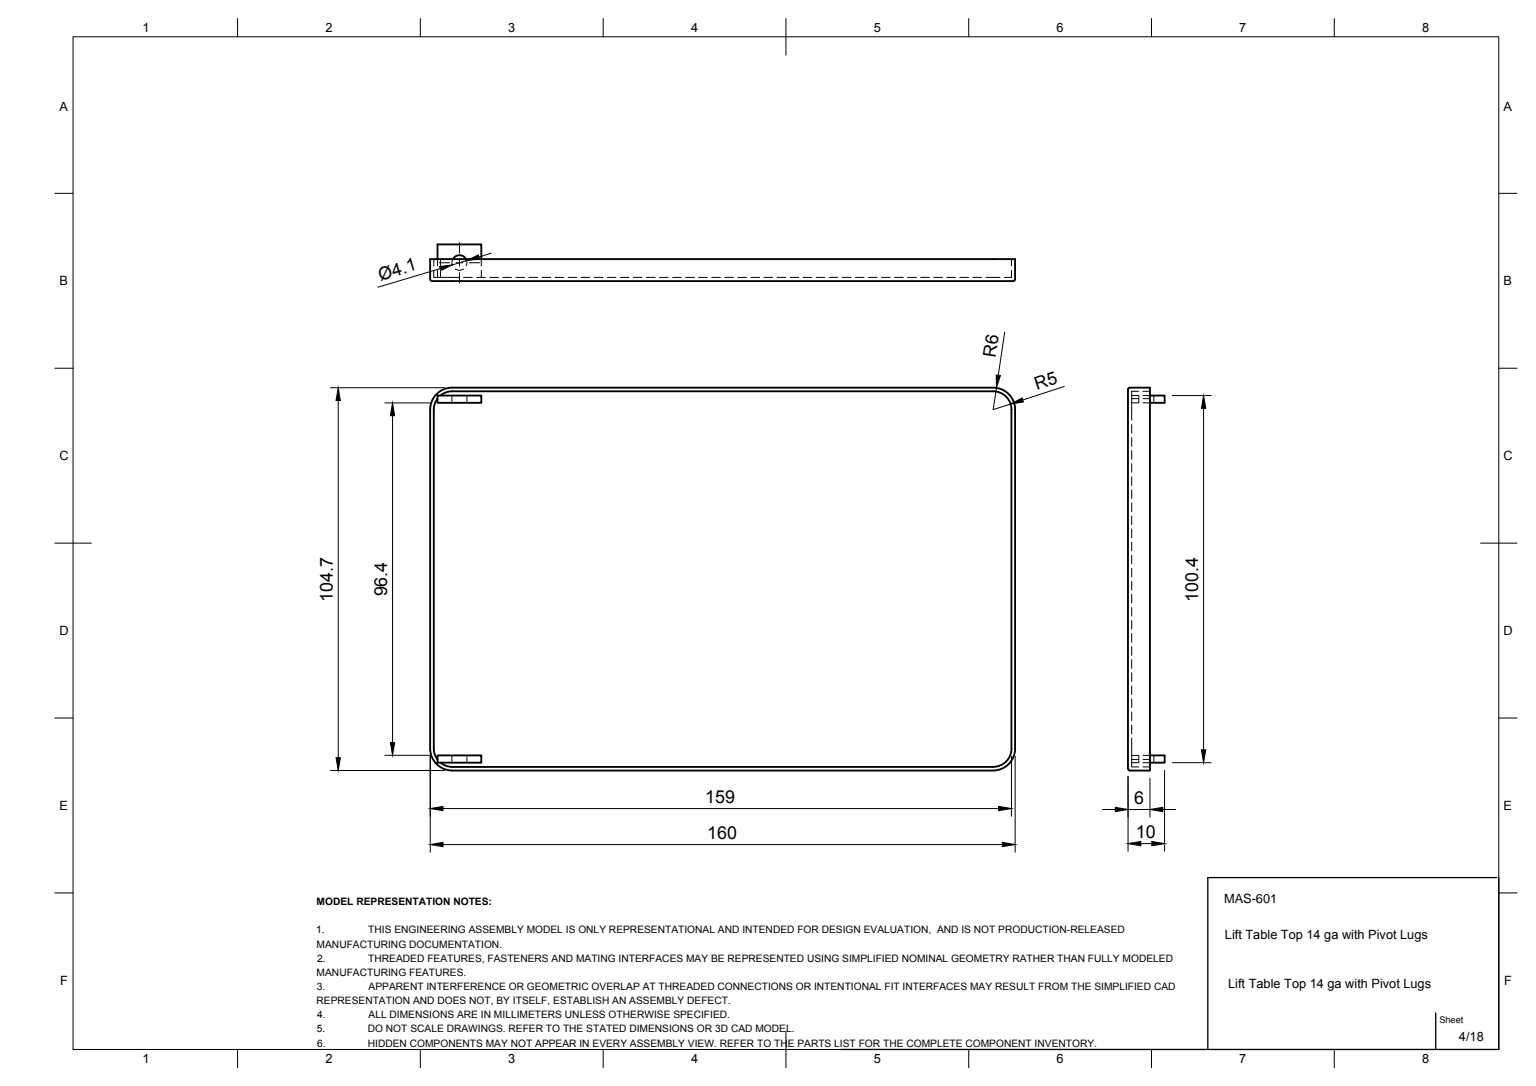
ISO-10303-21;
HEADER;
FILE_DESCRIPTION((''),'2;1');
FILE_NAME('Lift Table Top 14 ga with Pivot Lugs.step','2026-10-06T07:37:42+05:00',(''),(''),'','','');
FILE_SCHEMA (('AUTOMOTIVE_DESIGN { 1 0 10303 214 3 1 1 }'));
ENDSEC;
DATA;
#10=MECHANICAL_DESIGN_GEOMETRIC_PRESENTATION_REPRESENTATION('',(#374),#18757);
#331=TOROIDAL_SURFACE('',#9944,5.50000000000001,0.5) ;
#332=TOROIDAL_SURFACE('',#9950,5.50000000000001,0.5) ;
#333=TOROIDAL_SURFACE('',#9956,5.50000000000001,0.5) ;
#334=TOROIDAL_SURFACE('',#9962,5.50000000000001,0.5) ;
#340=SHAPE_REPRESENTATION_RELATIONSHIP('SRR','None',#18858,#357) ;
#357=ADVANCED_BREP_SHAPE_REPRESENTATION('',(#391),#18741) ;
#374=STYLED_ITEM('',(#18952),#391) ;
#391=MANIFOLD_SOLID_BREP('Lift Table Top 14 ga with Pivot Lugs',#9543) ;
#522=CYLINDRICAL_SURFACE('',#9906,2.05) ;
#523=CYLINDRICAL_SURFACE('',#9909,2.05) ;
#524=CYLINDRICAL_SURFACE('',#9917,5.00000000000001) ;
#525=CYLINDRICAL_SURFACE('',#9920,5.00000000000001) ;
#526=CYLINDRICAL_SURFACE('',#9937,5.00000000000001) ;
#527=CYLINDRICAL_SURFACE('',#9939,5.00000000000001) ;
#528=CYLINDRICAL_SURFACE('',#9941,0.5) ;
#529=CYLINDRICAL_SURFACE('',#9948,0.5) ;
#530=CYLINDRICAL_SURFACE('',#9954,0.5) ;
#531=CYLINDRICAL_SURFACE('',#9960,0.5) ;
#532=CYLINDRICAL_SURFACE('',#9965,6.00000000000001) ;
#533=CYLINDRICAL_SURFACE('',#9967,6.00000000000001) ;
#534=CYLINDRICAL_SURFACE('',#9971,5.00000000000001) ;
#535=CYLINDRICAL_SURFACE('',#9976,5.00000000000001) ;
#536=CYLINDRICAL_SURFACE('',#9979,6.00000000000001) ;
#537=CYLINDRICAL_SURFACE('',#9981,6.00000000000001) ;
#677=FACE_BOUND('',#1733,.T.) ;
#678=FACE_BOUND('',#1738,.T.) ;
#679=FACE_BOUND('',#1742,.T.) ;
#680=FACE_BOUND('',#1744,.T.) ;
#681=FACE_BOUND('',#1747,.T.) ;
#819=PLANE('',#9912) ;
#820=PLANE('',#9913) ;
#821=PLANE('',#9914) ;
#822=PLANE('',#9915) ;
#823=PLANE('',#9916) ;
#824=PLANE('',#9923) ;
#825=PLANE('',#9932) ;
#826=PLANE('',#9933) ;
#827=PLANE('',#9934) ;
#828=PLANE('',#9935) ;
#829=PLANE('',#9936) ;
#830=PLANE('',#9966) ;
#831=PLANE('',#9968) ;
#832=PLANE('',#9969) ;
#833=PLANE('',#9970) ;
#834=PLANE('',#9973) ;
#835=PLANE('',#9974) ;
#836=PLANE('',#9975) ;
#837=PLANE('',#9978) ;
#838=PLANE('',#9980) ;
#839=PLANE('',#9982) ;
#1185=FACE_OUTER_BOUND('',#1730,.T.) ;
#1186=FACE_OUTER_BOUND('',#1731,.T.) ;
#1187=FACE_OUTER_BOUND('',#1732,.T.) ;
#1188=FACE_OUTER_BOUND('',#1734,.T.) ;
#1189=FACE_OUTER_BOUND('',#1735,.T.) ;
#1190=FACE_OUTER_BOUND('',#1736,.T.) ;
#1191=FACE_OUTER_BOUND('',#1737,.T.) ;
#1192=FACE_OUTER_BOUND('',#1739,.T.) ;
#1193=FACE_OUTER_BOUND('',#1740,.T.) ;
#1194=FACE_OUTER_BOUND('',#1741,.T.) ;
#1195=FACE_OUTER_BOUND('',#1743,.T.) ;
#1196=FACE_OUTER_BOUND('',#1745,.T.) ;
#1197=FACE_OUTER_BOUND('',#1746,.T.) ;
#1198=FACE_OUTER_BOUND('',#1748,.T.) ;
#1199=FACE_OUTER_BOUND('',#1749,.T.) ;
#1200=FACE_OUTER_BOUND('',#1750,.T.) ;
#1201=FACE_OUTER_BOUND('',#1751,.T.) ;
#1202=FACE_OUTER_BOUND('',#1752,.T.) ;
#1203=FACE_OUTER_BOUND('',#1753,.T.) ;
#1204=FACE_OUTER_BOUND('',#1754,.T.) ;
#1205=FACE_OUTER_BOUND('',#1755,.T.) ;
#1206=FACE_OUTER_BOUND('',#1756,.T.) ;
#1207=FACE_OUTER_BOUND('',#1757,.T.) ;
#1208=FACE_OUTER_BOUND('',#1758,.T.) ;
#1209=FACE_OUTER_BOUND('',#1759,.T.) ;
#1210=FACE_OUTER_BOUND('',#1760,.T.) ;
#1211=FACE_OUTER_BOUND('',#1761,.T.) ;
#1212=FACE_OUTER_BOUND('',#1762,.T.) ;
#1213=FACE_OUTER_BOUND('',#1763,.T.) ;
#1214=FACE_OUTER_BOUND('',#1764,.T.) ;
#1215=FACE_OUTER_BOUND('',#1765,.T.) ;
#1216=FACE_OUTER_BOUND('',#1766,.T.) ;
#1217=FACE_OUTER_BOUND('',#1767,.T.) ;
#1218=FACE_OUTER_BOUND('',#1768,.T.) ;
#1219=FACE_OUTER_BOUND('',#1769,.T.) ;
#1220=FACE_OUTER_BOUND('',#1770,.T.) ;
#1221=FACE_OUTER_BOUND('',#1771,.T.) ;
#1222=FACE_OUTER_BOUND('',#1772,.T.) ;
#1223=FACE_OUTER_BOUND('',#1773,.T.) ;
#1224=FACE_OUTER_BOUND('',#1774,.T.) ;
#1225=FACE_OUTER_BOUND('',#1775,.T.) ;
#1730=EDGE_LOOP('',(#6859,#6860,#6861,#6862)) ;
#1731=EDGE_LOOP('',(#6863,#6864,#6865,#6866)) ;
#1732=EDGE_LOOP('',(#6867,#6868,#6869,#6870)) ;
#1733=EDGE_LOOP('',(#6871)) ;
#1734=EDGE_LOOP('',(#6872,#6873,#6874,#6875,#6876,#6877)) ;
#1735=EDGE_LOOP('',(#6878,#6879,#6880,#6881)) ;
#1736=EDGE_LOOP('',(#6882,#6883,#6884,#6885)) ;
#1737=EDGE_LOOP('',(#6886,#6887,#6888,#6889,#6890,#6891)) ;
#1738=EDGE_LOOP('',(#6892)) ;
#1739=EDGE_LOOP('',(#6893,#6894,#6895,#6896)) ;
#1740=EDGE_LOOP('',(#6897,#6898,#6899,#6900)) ;
#1741=EDGE_LOOP('',(#6901,#6902,#6903,#6904,#6905,#6906,#6907,#6908)) ;
#1742=EDGE_LOOP('',(#6909,#6910,#6911,#6912,#6913,#6914,#6915,#6916,#6917,
#6918,#6919,#6920,#6921,#6922)) ;
#1743=EDGE_LOOP('',(#6923,#6924,#6925,#6926)) ;
#1744=EDGE_LOOP('',(#6927)) ;
#1745=EDGE_LOOP('',(#6928,#6929,#6930,#6931)) ;
#1746=EDGE_LOOP('',(#6932,#6933,#6934,#6935,#6936,#6937)) ;
#1747=EDGE_LOOP('',(#6938)) ;
#1748=EDGE_LOOP('',(#6939,#6940,#6941,#6942)) ;
#1749=EDGE_LOOP('',(#6943,#6944,#6945,#6946,#6947,#6948)) ;
#1750=EDGE_LOOP('',(#6949,#6950,#6951,#6952)) ;
#1751=EDGE_LOOP('',(#6953,#6954,#6955,#6956)) ;
#1752=EDGE_LOOP('',(#6957,#6958,#6959,#6960)) ;
#1753=EDGE_LOOP('',(#6961,#6962,#6963,#6964)) ;
#1754=EDGE_LOOP('',(#6965,#6966,#6967,#6968)) ;
#1755=EDGE_LOOP('',(#6969,#6970,#6971,#6972)) ;
#1756=EDGE_LOOP('',(#6973,#6974,#6975,#6976)) ;
#1757=EDGE_LOOP('',(#6977,#6978,#6979,#6980)) ;
#1758=EDGE_LOOP('',(#6981,#6982,#6983,#6984)) ;
#1759=EDGE_LOOP('',(#6985,#6986,#6987,#6988)) ;
#1760=EDGE_LOOP('',(#6989,#6990,#6991,#6992)) ;
#1761=EDGE_LOOP('',(#6993,#6994,#6995,#6996)) ;
#1762=EDGE_LOOP('',(#6997,#6998,#6999,#7000)) ;
#1763=EDGE_LOOP('',(#7001,#7002,#7003,#7004)) ;
#1764=EDGE_LOOP('',(#7005,#7006,#7007,#7008,#7009,#7010,#7011,#7012)) ;
#1765=EDGE_LOOP('',(#7013,#7014,#7015,#7016)) ;
#1766=EDGE_LOOP('',(#7017,#7018,#7019,#7020)) ;
#1767=EDGE_LOOP('',(#7021,#7022,#7023,#7024)) ;
#1768=EDGE_LOOP('',(#7025,#7026,#7027,#7028)) ;
#1769=EDGE_LOOP('',(#7029,#7030,#7031,#7032)) ;
#1770=EDGE_LOOP('',(#7033,#7034,#7035,#7036)) ;
#1771=EDGE_LOOP('',(#7037,#7038,#7039,#7040,#7041,#7042,#7043,#7044,#7045,
#7046,#7047,#7048,#7049,#7050,#7051,#7052,#7053,#7054)) ;
#1772=EDGE_LOOP('',(#7055,#7056,#7057,#7058)) ;
#1773=EDGE_LOOP('',(#7059,#7060,#7061,#7062)) ;
#1774=EDGE_LOOP('',(#7063,#7064,#7065,#7066)) ;
#1775=EDGE_LOOP('',(#7067,#7068,#7069,#7070)) ;
#2421=LINE('',#14171,#3192) ;
#2422=LINE('',#14177,#3193) ;
#2423=LINE('',#14182,#3194) ;
#2424=LINE('',#14184,#3195) ;
#2425=LINE('',#14186,#3196) ;
#2426=LINE('',#14187,#3197) ;
#2427=LINE('',#14190,#3198) ;
#2428=LINE('',#14192,#3199) ;
#2429=LINE('',#14194,#3200) ;
#2430=LINE('',#14196,#3201) ;
#2431=LINE('',#14197,#3202) ;
#2432=LINE('',#14200,#3203) ;
#2433=LINE('',#14202,#3204) ;
#2434=LINE('',#14203,#3205) ;
#2435=LINE('',#14205,#3206) ;
#2436=LINE('',#14208,#3207) ;
#2437=LINE('',#14210,#3208) ;
#2438=LINE('',#14211,#3209) ;
#2439=LINE('',#14216,#3210) ;
#2440=LINE('',#14222,#3211) ;
#2441=LINE('',#14229,#3212) ;
#2442=LINE('',#14233,#3213) ;
#2443=LINE('',#14237,#3214) ;
#2444=LINE('',#14240,#3215) ;
#2445=LINE('',#14242,#3216) ;
#2446=LINE('',#14246,#3217) ;
#2447=LINE('',#14248,#3218) ;
#2448=LINE('',#14252,#3219) ;
#2449=LINE('',#14256,#3220) ;
#2450=LINE('',#14259,#3221) ;
#2451=LINE('',#14263,#3222) ;
#2452=LINE('',#14265,#3223) ;
#2453=LINE('',#14267,#3224) ;
#2454=LINE('',#14268,#3225) ;
#2455=LINE('',#14271,#3226) ;
#2456=LINE('',#14273,#3227) ;
#2457=LINE('',#14274,#3228) ;
#2458=LINE('',#14277,#3229) ;
#2459=LINE('',#14278,#3230) ;
#2460=LINE('',#14280,#3231) ;
#2461=LINE('',#14281,#3232) ;
#2462=LINE('',#14283,#3233) ;
#2463=LINE('',#14286,#3234) ;
#2464=LINE('',#14287,#3235) ;
#2465=LINE('',#14291,#3236) ;
#2466=LINE('',#14294,#3237) ;
#2467=LINE('',#14301,#3238) ;
#2468=LINE('',#14304,#3239) ;
#2469=LINE('',#14315,#3240) ;
#2470=LINE('',#14316,#3241) ;
#2471=LINE('',#14327,#3242) ;
#2472=LINE('',#14328,#3243) ;
#2473=LINE('',#14339,#3244) ;
#2474=LINE('',#14340,#3245) ;
#2475=LINE('',#14345,#3246) ;
#2476=LINE('',#14346,#3247) ;
#2477=LINE('',#14348,#3248) ;
#2478=LINE('',#14350,#3249) ;
#2479=LINE('',#14352,#3250) ;
#2480=LINE('',#14356,#3251) ;
#2481=LINE('',#14358,#3252) ;
#2482=LINE('',#14359,#3253) ;
#2483=LINE('',#14362,#3254) ;
#2484=LINE('',#14365,#3255) ;
#2485=LINE('',#14367,#3256) ;
#2486=LINE('',#14370,#3257) ;
#2487=LINE('',#14371,#3258) ;
#2488=LINE('',#14376,#3259) ;
#2489=LINE('',#14378,#3260) ;
#2490=LINE('',#14380,#3261) ;
#3192=VECTOR('',#11225,2.05) ;
#3193=VECTOR('',#11232,2.05) ;
#3194=VECTOR('',#11237,10.) ;
#3195=VECTOR('',#11238,10.) ;
#3196=VECTOR('',#11239,10.) ;
#3197=VECTOR('',#11240,10.) ;
#3198=VECTOR('',#11243,10.) ;
#3199=VECTOR('',#11244,10.) ;
#3200=VECTOR('',#11245,10.) ;
#3201=VECTOR('',#11246,10.) ;
#3202=VECTOR('',#11247,10.) ;
#3203=VECTOR('',#11250,10.) ;
#3204=VECTOR('',#11251,10.) ;
#3205=VECTOR('',#11252,10.) ;
#3206=VECTOR('',#11255,10.) ;
#3207=VECTOR('',#11258,10.) ;
#3208=VECTOR('',#11259,10.) ;
#3209=VECTOR('',#11260,10.) ;
#3210=VECTOR('',#11265,10.) ;
#3211=VECTOR('',#11272,10.) ;
#3212=VECTOR('',#11279,10.) ;
#3213=VECTOR('',#11282,10.) ;
#3214=VECTOR('',#11285,10.) ;
#3215=VECTOR('',#11288,10.) ;
#3216=VECTOR('',#11289,10.) ;
#3217=VECTOR('',#11292,10.) ;
#3218=VECTOR('',#11293,10.) ;
#3219=VECTOR('',#11296,10.) ;
#3220=VECTOR('',#11299,10.) ;
#3221=VECTOR('',#11302,10.) ;
#3222=VECTOR('',#11305,10.) ;
#3223=VECTOR('',#11306,10.) ;
#3224=VECTOR('',#11307,10.) ;
#3225=VECTOR('',#11308,10.) ;
#3226=VECTOR('',#11311,10.) ;
#3227=VECTOR('',#11312,10.) ;
#3228=VECTOR('',#11313,10.) ;
#3229=VECTOR('',#11316,10.) ;
#3230=VECTOR('',#11317,10.) ;
#3231=VECTOR('',#11318,10.) ;
#3232=VECTOR('',#11319,10.) ;
#3233=VECTOR('',#11322,10.) ;
#3234=VECTOR('',#11325,10.) ;
#3235=VECTOR('',#11326,10.) ;
#3236=VECTOR('',#11331,10.) ;
#3237=VECTOR('',#11334,10.) ;
#3238=VECTOR('',#11341,10.) ;
#3239=VECTOR('',#11344,10.) ;
#3240=VECTOR('',#11357,10.) ;
#3241=VECTOR('',#11358,10.) ;
#3242=VECTOR('',#11371,10.) ;
#3243=VECTOR('',#11372,10.) ;
#3244=VECTOR('',#11385,10.) ;
#3245=VECTOR('',#11386,10.) ;
#3246=VECTOR('',#11395,10.) ;
#3247=VECTOR('',#11396,10.) ;
#3248=VECTOR('',#11399,10.) ;
#3249=VECTOR('',#11402,10.) ;
#3250=VECTOR('',#11405,10.) ;
#3251=VECTOR('',#11410,10.) ;
#3252=VECTOR('',#11411,10.) ;
#3253=VECTOR('',#11412,10.) ;
#3254=VECTOR('',#11415,10.) ;
#3255=VECTOR('',#11420,10.) ;
#3256=VECTOR('',#11423,10.) ;
#3257=VECTOR('',#11426,10.) ;
#3258=VECTOR('',#11427,10.) ;
#3259=VECTOR('',#11436,10.) ;
#3260=VECTOR('',#11439,10.) ;
#3261=VECTOR('',#11442,10.) ;
#3833=CIRCLE('',#9907,2.05) ;
#3834=CIRCLE('',#9908,2.05) ;
#3835=CIRCLE('',#9910,2.05) ;
#3836=CIRCLE('',#9911,2.05) ;
#3837=CIRCLE('',#9918,5.00000000000001) ;
#3838=CIRCLE('',#9919,5.00000000000001) ;
#3839=CIRCLE('',#9921,5.00000000000001) ;
#3840=CIRCLE('',#9922,5.00000000000001) ;
#3841=CIRCLE('',#9924,6.00000000000001) ;
#3842=CIRCLE('',#9925,6.00000000000001) ;
#3843=CIRCLE('',#9926,6.00000000000001) ;
#3844=CIRCLE('',#9927,6.00000000000001) ;
#3845=CIRCLE('',#9928,5.00000000000001) ;
#3846=CIRCLE('',#9929,5.00000000000001) ;
#3847=CIRCLE('',#9930,5.00000000000001) ;
#3848=CIRCLE('',#9931,5.00000000000001) ;
#3849=CIRCLE('',#9938,5.00000000000001) ;
#3850=CIRCLE('',#9940,5.00000000000001) ;
#3851=CIRCLE('',#9942,0.499999999999989) ;
#3852=CIRCLE('',#9943,0.499999999999998) ;
#3853=CIRCLE('',#9945,0.500000000000007) ;
#3854=CIRCLE('',#9946,5.50000000000001) ;
#3855=CIRCLE('',#9947,6.00000000000002) ;
#3856=CIRCLE('',#9949,0.499999999999998) ;
#3857=CIRCLE('',#9951,0.499999999999998) ;
#3858=CIRCLE('',#9952,5.50000000000001) ;
#3859=CIRCLE('',#9953,6.00000000000002) ;
#3860=CIRCLE('',#9955,0.499999999999998) ;
#3861=CIRCLE('',#9957,0.500000000000007) ;
#3862=CIRCLE('',#9958,5.50000000000001) ;
#3863=CIRCLE('',#9959,6.00000000000002) ;
#3864=CIRCLE('',#9961,0.499999999999998) ;
#3865=CIRCLE('',#9963,5.50000000000001) ;
#3866=CIRCLE('',#9964,6.00000000000002) ;
#3867=CIRCLE('',#9972,5.00000000000001) ;
#3868=CIRCLE('',#9977,5.00000000000001) ;
#4320=VERTEX_POINT('',#14168) ;
#4321=VERTEX_POINT('',#14170) ;
#4322=VERTEX_POINT('',#14174) ;
#4323=VERTEX_POINT('',#14176) ;
#4324=VERTEX_POINT('',#14180) ;
#4325=VERTEX_POINT('',#14181) ;
#4326=VERTEX_POINT('',#14183) ;
#4327=VERTEX_POINT('',#14185) ;
#4328=VERTEX_POINT('',#14189) ;
#4329=VERTEX_POINT('',#14191) ;
#4330=VERTEX_POINT('',#14193) ;
#4331=VERTEX_POINT('',#14195) ;
#4332=VERTEX_POINT('',#14199) ;
#4333=VERTEX_POINT('',#14201) ;
#4334=VERTEX_POINT('',#14207) ;
#4335=VERTEX_POINT('',#14209) ;
#4336=VERTEX_POINT('',#14213) ;
#4337=VERTEX_POINT('',#14215) ;
#4338=VERTEX_POINT('',#14219) ;
#4339=VERTEX_POINT('',#14221) ;
#4340=VERTEX_POINT('',#14225) ;
#4341=VERTEX_POINT('',#14226) ;
#4342=VERTEX_POINT('',#14228) ;
#4343=VERTEX_POINT('',#14230) ;
#4344=VERTEX_POINT('',#14232) ;
#4345=VERTEX_POINT('',#14234) ;
#4346=VERTEX_POINT('',#14236) ;
#4347=VERTEX_POINT('',#14238) ;
#4348=VERTEX_POINT('',#14241) ;
#4349=VERTEX_POINT('',#14243) ;
#4350=VERTEX_POINT('',#14245) ;
#4351=VERTEX_POINT('',#14247) ;
#4352=VERTEX_POINT('',#14249) ;
#4353=VERTEX_POINT('',#14251) ;
#4354=VERTEX_POINT('',#14253) ;
#4355=VERTEX_POINT('',#14255) ;
#4356=VERTEX_POINT('',#14257) ;
#4357=VERTEX_POINT('',#14261) ;
#4358=VERTEX_POINT('',#14262) ;
#4359=VERTEX_POINT('',#14264) ;
#4360=VERTEX_POINT('',#14266) ;
#4361=VERTEX_POINT('',#14270) ;
#4362=VERTEX_POINT('',#14272) ;
#4363=VERTEX_POINT('',#14276) ;
#4364=VERTEX_POINT('',#14279) ;
#4365=VERTEX_POINT('',#14285) ;
#4366=VERTEX_POINT('',#14289) ;
#4367=VERTEX_POINT('',#14293) ;
#4368=VERTEX_POINT('',#14297) ;
#4369=VERTEX_POINT('',#14298) ;
#4370=VERTEX_POINT('',#14300) ;
#4371=VERTEX_POINT('',#14302) ;
#4372=VERTEX_POINT('',#14306) ;
#4373=VERTEX_POINT('',#14307) ;
#4374=VERTEX_POINT('',#14312) ;
#4375=VERTEX_POINT('',#14313) ;
#4376=VERTEX_POINT('',#14318) ;
#4377=VERTEX_POINT('',#14319) ;
#4378=VERTEX_POINT('',#14324) ;
#4379=VERTEX_POINT('',#14325) ;
#4380=VERTEX_POINT('',#14330) ;
#4381=VERTEX_POINT('',#14331) ;
#4382=VERTEX_POINT('',#14336) ;
#4383=VERTEX_POINT('',#14337) ;
#4384=VERTEX_POINT('',#14355) ;
#4385=VERTEX_POINT('',#14357) ;
#4386=VERTEX_POINT('',#14361) ;
#4387=VERTEX_POINT('',#14369) ;
#5276=EDGE_CURVE('',#4320,#4320,#3833,.T.) ;
#5277=EDGE_CURVE('',#4320,#4321,#2421,.T.) ;
#5278=EDGE_CURVE('',#4321,#4321,#3834,.T.) ;
#5279=EDGE_CURVE('',#4322,#4322,#3835,.T.) ;
#5280=EDGE_CURVE('',#4322,#4323,#2422,.T.) ;
#5281=EDGE_CURVE('',#4323,#4323,#3836,.T.) ;
#5282=EDGE_CURVE('',#4324,#4325,#2423,.T.) ;
#5283=EDGE_CURVE('',#4324,#4326,#2424,.T.) ;
#5284=EDGE_CURVE('',#4326,#4327,#2425,.T.) ;
#5285=EDGE_CURVE('',#4327,#4325,#2426,.T.) ;
#5286=EDGE_CURVE('',#4328,#4324,#2427,.T.) ;
#5287=EDGE_CURVE('',#4329,#4328,#2428,.T.) ;
#5288=EDGE_CURVE('',#4330,#4329,#2429,.T.) ;
#5289=EDGE_CURVE('',#4331,#4330,#2430,.T.) ;
#5290=EDGE_CURVE('',#4331,#4326,#2431,.T.) ;
#5291=EDGE_CURVE('',#4325,#4332,#2432,.T.) ;
#5292=EDGE_CURVE('',#4333,#4327,#2433,.T.) ;
#5293=EDGE_CURVE('',#4332,#4333,#2434,.T.) ;
#5294=EDGE_CURVE('',#4333,#4331,#2435,.T.) ;
#5295=EDGE_CURVE('',#4332,#4334,#2436,.T.) ;
#5296=EDGE_CURVE('',#4335,#4330,#2437,.T.) ;
#5297=EDGE_CURVE('',#4334,#4335,#2438,.T.) ;
#5298=EDGE_CURVE('',#4328,#4336,#3837,.T.) ;
#5299=EDGE_CURVE('',#4337,#4336,#2439,.T.) ;
#5300=EDGE_CURVE('',#4329,#4337,#3838,.T.) ;
#5301=EDGE_CURVE('',#4338,#4335,#3839,.T.) ;
#5302=EDGE_CURVE('',#4338,#4339,#2440,.T.) ;
#5303=EDGE_CURVE('',#4339,#4334,#3840,.T.) ;
#5304=EDGE_CURVE('',#4340,#4341,#3841,.T.) ;
#5305=EDGE_CURVE('',#4342,#4340,#2441,.T.) ;
#5306=EDGE_CURVE('',#4343,#4342,#3842,.T.) ;
#5307=EDGE_CURVE('',#4344,#4343,#2442,.T.) ;
#5308=EDGE_CURVE('',#4345,#4344,#3843,.T.) ;
#5309=EDGE_CURVE('',#4346,#4345,#2443,.T.) ;
#5310=EDGE_CURVE('',#4347,#4346,#3844,.T.) ;
#5311=EDGE_CURVE('',#4341,#4347,#2444,.T.) ;
#5312=EDGE_CURVE('',#4337,#4348,#2445,.T.) ;
#5313=EDGE_CURVE('',#4348,#4349,#3845,.T.) ;
#5314=EDGE_CURVE('',#4349,#4350,#2446,.T.) ;
#5315=EDGE_CURVE('',#4350,#4351,#2447,.T.) ;
#5316=EDGE_CURVE('',#4351,#4352,#3846,.T.) ;
#5317=EDGE_CURVE('',#4352,#4353,#2448,.T.) ;
#5318=EDGE_CURVE('',#4353,#4354,#3847,.T.) ;
#5319=EDGE_CURVE('',#4354,#4355,#2449,.T.) ;
#5320=EDGE_CURVE('',#4355,#4356,#3848,.T.) ;
#5321=EDGE_CURVE('',#4356,#4338,#2450,.T.) ;
#5322=EDGE_CURVE('',#4357,#4358,#2451,.T.) ;
#5323=EDGE_CURVE('',#4357,#4359,#2452,.T.) ;
#5324=EDGE_CURVE('',#4359,#4360,#2453,.T.) ;
#5325=EDGE_CURVE('',#4360,#4358,#2454,.T.) ;
#5326=EDGE_CURVE('',#4361,#4357,#2455,.T.) ;
#5327=EDGE_CURVE('',#4362,#4361,#2456,.T.) ;
#5328=EDGE_CURVE('',#4359,#4362,#2457,.T.) ;
#5329=EDGE_CURVE('',#4363,#4361,#2458,.T.) ;
#5330=EDGE_CURVE('',#4351,#4363,#2459,.T.) ;
#5331=EDGE_CURVE('',#4350,#4364,#2460,.T.) ;
#5332=EDGE_CURVE('',#4364,#4362,#2461,.T.) ;
#5333=EDGE_CURVE('',#4360,#4364,#2462,.T.) ;
#5334=EDGE_CURVE('',#4358,#4365,#2463,.T.) ;
#5335=EDGE_CURVE('',#4365,#4349,#2464,.T.) ;
#5336=EDGE_CURVE('',#4363,#4366,#3849,.T.) ;
#5337=EDGE_CURVE('',#4352,#4366,#2465,.T.) ;
#5338=EDGE_CURVE('',#4348,#4367,#2466,.T.) ;
#5339=EDGE_CURVE('',#4367,#4365,#3850,.T.) ;
#5340=EDGE_CURVE('',#4368,#4369,#3851,.T.) ;
#5341=EDGE_CURVE('',#4369,#4370,#2467,.T.) ;
#5342=EDGE_CURVE('',#4370,#4371,#3852,.T.) ;
#5343=EDGE_CURVE('',#4371,#4368,#2468,.T.) ;
#5344=EDGE_CURVE('',#4372,#4373,#3853,.T.) ;
#5345=EDGE_CURVE('',#4373,#4371,#3854,.T.) ;
#5346=EDGE_CURVE('',#4370,#4372,#3855,.T.) ;
#5347=EDGE_CURVE('',#4374,#4375,#3856,.T.) ;
#5348=EDGE_CURVE('',#4375,#4373,#2469,.T.) ;
#5349=EDGE_CURVE('',#4372,#4374,#2470,.T.) ;
#5350=EDGE_CURVE('',#4376,#4377,#3857,.T.) ;
#5351=EDGE_CURVE('',#4377,#4375,#3858,.T.) ;
#5352=EDGE_CURVE('',#4374,#4376,#3859,.T.) ;
#5353=EDGE_CURVE('',#4378,#4379,#3860,.T.) ;
#5354=EDGE_CURVE('',#4379,#4377,#2471,.T.) ;
#5355=EDGE_CURVE('',#4376,#4378,#2472,.T.) ;
#5356=EDGE_CURVE('',#4380,#4381,#3861,.T.) ;
#5357=EDGE_CURVE('',#4381,#4379,#3862,.T.) ;
#5358=EDGE_CURVE('',#4378,#4380,#3863,.T.) ;
#5359=EDGE_CURVE('',#4382,#4383,#3864,.T.) ;
#5360=EDGE_CURVE('',#4383,#4381,#2473,.T.) ;
#5361=EDGE_CURVE('',#4380,#4382,#2474,.T.) ;
#5362=EDGE_CURVE('',#4368,#4383,#3865,.T.) ;
#5363=EDGE_CURVE('',#4382,#4369,#3866,.T.) ;
#5364=EDGE_CURVE('',#4347,#4374,#2475,.T.) ;
#5365=EDGE_CURVE('',#4346,#4376,#2476,.T.) ;
#5366=EDGE_CURVE('',#4341,#4372,#2477,.T.) ;
#5367=EDGE_CURVE('',#4340,#4370,#2478,.T.) ;
#5368=EDGE_CURVE('',#4342,#4369,#2479,.T.) ;
#5369=EDGE_CURVE('',#4354,#4384,#2480,.T.) ;
#5370=EDGE_CURVE('',#4384,#4385,#2481,.T.) ;
#5371=EDGE_CURVE('',#4355,#4385,#2482,.T.) ;
#5372=EDGE_CURVE('',#4353,#4386,#2483,.T.) ;
#5373=EDGE_CURVE('',#4386,#4384,#3867,.T.) ;
#5374=EDGE_CURVE('',#4366,#4386,#2484,.T.) ;
#5375=EDGE_CURVE('',#4336,#4367,#2485,.T.) ;
#5376=EDGE_CURVE('',#4356,#4387,#2486,.T.) ;
#5377=EDGE_CURVE('',#4387,#4339,#2487,.T.) ;
#5378=EDGE_CURVE('',#4385,#4387,#3868,.T.) ;
#5379=EDGE_CURVE('',#4343,#4382,#2488,.T.) ;
#5380=EDGE_CURVE('',#4344,#4380,#2489,.T.) ;
#5381=EDGE_CURVE('',#4345,#4378,#2490,.T.) ;
#6859=ORIENTED_EDGE('',*,*,#5276,.F.) ;
#6860=ORIENTED_EDGE('',*,*,#5277,.T.) ;
#6861=ORIENTED_EDGE('',*,*,#5278,.F.) ;
#6862=ORIENTED_EDGE('',*,*,#5277,.F.) ;
#6863=ORIENTED_EDGE('',*,*,#5279,.F.) ;
#6864=ORIENTED_EDGE('',*,*,#5280,.T.) ;
#6865=ORIENTED_EDGE('',*,*,#5281,.F.) ;
#6866=ORIENTED_EDGE('',*,*,#5280,.F.) ;
#6867=ORIENTED_EDGE('',*,*,#5282,.F.) ;
#6868=ORIENTED_EDGE('',*,*,#5283,.T.) ;
#6869=ORIENTED_EDGE('',*,*,#5284,.T.) ;
#6870=ORIENTED_EDGE('',*,*,#5285,.T.) ;
#6871=ORIENTED_EDGE('',*,*,#5281,.T.) ;
#6872=ORIENTED_EDGE('',*,*,#5286,.F.) ;
#6873=ORIENTED_EDGE('',*,*,#5287,.F.) ;
#6874=ORIENTED_EDGE('',*,*,#5288,.F.) ;
#6875=ORIENTED_EDGE('',*,*,#5289,.F.) ;
#6876=ORIENTED_EDGE('',*,*,#5290,.T.) ;
#6877=ORIENTED_EDGE('',*,*,#5283,.F.) ;
#6878=ORIENTED_EDGE('',*,*,#5291,.F.) ;
#6879=ORIENTED_EDGE('',*,*,#5285,.F.) ;
#6880=ORIENTED_EDGE('',*,*,#5292,.F.) ;
#6881=ORIENTED_EDGE('',*,*,#5293,.F.) ;
#6882=ORIENTED_EDGE('',*,*,#5294,.F.) ;
#6883=ORIENTED_EDGE('',*,*,#5292,.T.) ;
#6884=ORIENTED_EDGE('',*,*,#5284,.F.) ;
#6885=ORIENTED_EDGE('',*,*,#5290,.F.) ;
#6886=ORIENTED_EDGE('',*,*,#5295,.F.) ;
#6887=ORIENTED_EDGE('',*,*,#5293,.T.) ;
#6888=ORIENTED_EDGE('',*,*,#5294,.T.) ;
#6889=ORIENTED_EDGE('',*,*,#5289,.T.) ;
#6890=ORIENTED_EDGE('',*,*,#5296,.F.) ;
#6891=ORIENTED_EDGE('',*,*,#5297,.F.) ;
#6892=ORIENTED_EDGE('',*,*,#5279,.T.) ;
#6893=ORIENTED_EDGE('',*,*,#5287,.T.) ;
#6894=ORIENTED_EDGE('',*,*,#5298,.T.) ;
#6895=ORIENTED_EDGE('',*,*,#5299,.F.) ;
#6896=ORIENTED_EDGE('',*,*,#5300,.F.) ;
#6897=ORIENTED_EDGE('',*,*,#5297,.T.) ;
#6898=ORIENTED_EDGE('',*,*,#5301,.F.) ;
#6899=ORIENTED_EDGE('',*,*,#5302,.T.) ;
#6900=ORIENTED_EDGE('',*,*,#5303,.T.) ;
#6901=ORIENTED_EDGE('',*,*,#5304,.F.) ;
#6902=ORIENTED_EDGE('',*,*,#5305,.F.) ;
#6903=ORIENTED_EDGE('',*,*,#5306,.F.) ;
#6904=ORIENTED_EDGE('',*,*,#5307,.F.) ;
#6905=ORIENTED_EDGE('',*,*,#5308,.F.) ;
#6906=ORIENTED_EDGE('',*,*,#5309,.F.) ;
#6907=ORIENTED_EDGE('',*,*,#5310,.F.) ;
#6908=ORIENTED_EDGE('',*,*,#5311,.F.) ;
#6909=ORIENTED_EDGE('',*,*,#5296,.T.) ;
#6910=ORIENTED_EDGE('',*,*,#5288,.T.) ;
#6911=ORIENTED_EDGE('',*,*,#5300,.T.) ;
#6912=ORIENTED_EDGE('',*,*,#5312,.T.) ;
#6913=ORIENTED_EDGE('',*,*,#5313,.T.) ;
#6914=ORIENTED_EDGE('',*,*,#5314,.T.) ;
#6915=ORIENTED_EDGE('',*,*,#5315,.T.) ;
#6916=ORIENTED_EDGE('',*,*,#5316,.T.) ;
#6917=ORIENTED_EDGE('',*,*,#5317,.T.) ;
#6918=ORIENTED_EDGE('',*,*,#5318,.T.) ;
#6919=ORIENTED_EDGE('',*,*,#5319,.T.) ;
#6920=ORIENTED_EDGE('',*,*,#5320,.T.) ;
#6921=ORIENTED_EDGE('',*,*,#5321,.T.) ;
#6922=ORIENTED_EDGE('',*,*,#5301,.T.) ;
#6923=ORIENTED_EDGE('',*,*,#5322,.F.) ;
#6924=ORIENTED_EDGE('',*,*,#5323,.T.) ;
#6925=ORIENTED_EDGE('',*,*,#5324,.T.) ;
#6926=ORIENTED_EDGE('',*,*,#5325,.T.) ;
#6927=ORIENTED_EDGE('',*,*,#5276,.T.) ;
#6928=ORIENTED_EDGE('',*,*,#5326,.F.) ;
#6929=ORIENTED_EDGE('',*,*,#5327,.F.) ;
#6930=ORIENTED_EDGE('',*,*,#5328,.F.) ;
#6931=ORIENTED_EDGE('',*,*,#5323,.F.) ;
#6932=ORIENTED_EDGE('',*,*,#5329,.F.) ;
#6933=ORIENTED_EDGE('',*,*,#5330,.F.) ;
#6934=ORIENTED_EDGE('',*,*,#5315,.F.) ;
#6935=ORIENTED_EDGE('',*,*,#5331,.T.) ;
#6936=ORIENTED_EDGE('',*,*,#5332,.T.) ;
#6937=ORIENTED_EDGE('',*,*,#5327,.T.) ;
#6938=ORIENTED_EDGE('',*,*,#5278,.T.) ;
#6939=ORIENTED_EDGE('',*,*,#5324,.F.) ;
#6940=ORIENTED_EDGE('',*,*,#5328,.T.) ;
#6941=ORIENTED_EDGE('',*,*,#5332,.F.) ;
#6942=ORIENTED_EDGE('',*,*,#5333,.F.) ;
#6943=ORIENTED_EDGE('',*,*,#5334,.F.) ;
#6944=ORIENTED_EDGE('',*,*,#5325,.F.) ;
#6945=ORIENTED_EDGE('',*,*,#5333,.T.) ;
#6946=ORIENTED_EDGE('',*,*,#5331,.F.) ;
#6947=ORIENTED_EDGE('',*,*,#5314,.F.) ;
#6948=ORIENTED_EDGE('',*,*,#5335,.F.) ;
#6949=ORIENTED_EDGE('',*,*,#5330,.T.) ;
#6950=ORIENTED_EDGE('',*,*,#5336,.T.) ;
#6951=ORIENTED_EDGE('',*,*,#5337,.F.) ;
#6952=ORIENTED_EDGE('',*,*,#5316,.F.) ;
#6953=ORIENTED_EDGE('',*,*,#5335,.T.) ;
#6954=ORIENTED_EDGE('',*,*,#5313,.F.) ;
#6955=ORIENTED_EDGE('',*,*,#5338,.T.) ;
#6956=ORIENTED_EDGE('',*,*,#5339,.T.) ;
#6957=ORIENTED_EDGE('',*,*,#5340,.T.) ;
#6958=ORIENTED_EDGE('',*,*,#5341,.T.) ;
#6959=ORIENTED_EDGE('',*,*,#5342,.T.) ;
#6960=ORIENTED_EDGE('',*,*,#5343,.T.) ;
#6961=ORIENTED_EDGE('',*,*,#5344,.T.) ;
#6962=ORIENTED_EDGE('',*,*,#5345,.T.) ;
#6963=ORIENTED_EDGE('',*,*,#5342,.F.) ;
#6964=ORIENTED_EDGE('',*,*,#5346,.T.) ;
#6965=ORIENTED_EDGE('',*,*,#5347,.T.) ;
#6966=ORIENTED_EDGE('',*,*,#5348,.T.) ;
#6967=ORIENTED_EDGE('',*,*,#5344,.F.) ;
#6968=ORIENTED_EDGE('',*,*,#5349,.T.) ;
#6969=ORIENTED_EDGE('',*,*,#5350,.T.) ;
#6970=ORIENTED_EDGE('',*,*,#5351,.T.) ;
#6971=ORIENTED_EDGE('',*,*,#5347,.F.) ;
#6972=ORIENTED_EDGE('',*,*,#5352,.T.) ;
#6973=ORIENTED_EDGE('',*,*,#5353,.T.) ;
#6974=ORIENTED_EDGE('',*,*,#5354,.T.) ;
#6975=ORIENTED_EDGE('',*,*,#5350,.F.) ;
#6976=ORIENTED_EDGE('',*,*,#5355,.T.) ;
#6977=ORIENTED_EDGE('',*,*,#5356,.T.) ;
#6978=ORIENTED_EDGE('',*,*,#5357,.T.) ;
#6979=ORIENTED_EDGE('',*,*,#5353,.F.) ;
#6980=ORIENTED_EDGE('',*,*,#5358,.T.) ;
#6981=ORIENTED_EDGE('',*,*,#5359,.T.) ;
#6982=ORIENTED_EDGE('',*,*,#5360,.T.) ;
#6983=ORIENTED_EDGE('',*,*,#5356,.F.) ;
#6984=ORIENTED_EDGE('',*,*,#5361,.T.) ;
#6985=ORIENTED_EDGE('',*,*,#5340,.F.) ;
#6986=ORIENTED_EDGE('',*,*,#5362,.T.) ;
#6987=ORIENTED_EDGE('',*,*,#5359,.F.) ;
#6988=ORIENTED_EDGE('',*,*,#5363,.T.) ;
#6989=ORIENTED_EDGE('',*,*,#5352,.F.) ;
#6990=ORIENTED_EDGE('',*,*,#5364,.F.) ;
#6991=ORIENTED_EDGE('',*,*,#5310,.T.) ;
#6992=ORIENTED_EDGE('',*,*,#5365,.T.) ;
#6993=ORIENTED_EDGE('',*,*,#5349,.F.) ;
#6994=ORIENTED_EDGE('',*,*,#5366,.F.) ;
#6995=ORIENTED_EDGE('',*,*,#5311,.T.) ;
#6996=ORIENTED_EDGE('',*,*,#5364,.T.) ;
#6997=ORIENTED_EDGE('',*,*,#5346,.F.) ;
#6998=ORIENTED_EDGE('',*,*,#5367,.F.) ;
#6999=ORIENTED_EDGE('',*,*,#5304,.T.) ;
#7000=ORIENTED_EDGE('',*,*,#5366,.T.) ;
#7001=ORIENTED_EDGE('',*,*,#5341,.F.) ;
#7002=ORIENTED_EDGE('',*,*,#5368,.F.) ;
#7003=ORIENTED_EDGE('',*,*,#5305,.T.) ;
#7004=ORIENTED_EDGE('',*,*,#5367,.T.) ;
#7005=ORIENTED_EDGE('',*,*,#5343,.F.) ;
#7006=ORIENTED_EDGE('',*,*,#5345,.F.) ;
#7007=ORIENTED_EDGE('',*,*,#5348,.F.) ;
#7008=ORIENTED_EDGE('',*,*,#5351,.F.) ;
#7009=ORIENTED_EDGE('',*,*,#5354,.F.) ;
#7010=ORIENTED_EDGE('',*,*,#5357,.F.) ;
#7011=ORIENTED_EDGE('',*,*,#5360,.F.) ;
#7012=ORIENTED_EDGE('',*,*,#5362,.F.) ;
#7013=ORIENTED_EDGE('',*,*,#5319,.F.) ;
#7014=ORIENTED_EDGE('',*,*,#5369,.T.) ;
#7015=ORIENTED_EDGE('',*,*,#5370,.T.) ;
#7016=ORIENTED_EDGE('',*,*,#5371,.F.) ;
#7017=ORIENTED_EDGE('',*,*,#5318,.F.) ;
#7018=ORIENTED_EDGE('',*,*,#5372,.T.) ;
#7019=ORIENTED_EDGE('',*,*,#5373,.T.) ;
#7020=ORIENTED_EDGE('',*,*,#5369,.F.) ;
#7021=ORIENTED_EDGE('',*,*,#5317,.F.) ;
#7022=ORIENTED_EDGE('',*,*,#5337,.T.) ;
#7023=ORIENTED_EDGE('',*,*,#5374,.T.) ;
#7024=ORIENTED_EDGE('',*,*,#5372,.F.) ;
#7025=ORIENTED_EDGE('',*,*,#5312,.F.) ;
#7026=ORIENTED_EDGE('',*,*,#5299,.T.) ;
#7027=ORIENTED_EDGE('',*,*,#5375,.T.) ;
#7028=ORIENTED_EDGE('',*,*,#5338,.F.) ;
#7029=ORIENTED_EDGE('',*,*,#5321,.F.) ;
#7030=ORIENTED_EDGE('',*,*,#5376,.T.) ;
#7031=ORIENTED_EDGE('',*,*,#5377,.T.) ;
#7032=ORIENTED_EDGE('',*,*,#5302,.F.) ;
#7033=ORIENTED_EDGE('',*,*,#5320,.F.) ;
#7034=ORIENTED_EDGE('',*,*,#5371,.T.) ;
#7035=ORIENTED_EDGE('',*,*,#5378,.T.) ;
#7036=ORIENTED_EDGE('',*,*,#5376,.F.) ;
#7037=ORIENTED_EDGE('',*,*,#5295,.T.) ;
#7038=ORIENTED_EDGE('',*,*,#5303,.F.) ;
#7039=ORIENTED_EDGE('',*,*,#5377,.F.) ;
#7040=ORIENTED_EDGE('',*,*,#5378,.F.) ;
#7041=ORIENTED_EDGE('',*,*,#5370,.F.) ;
#7042=ORIENTED_EDGE('',*,*,#5373,.F.) ;
#7043=ORIENTED_EDGE('',*,*,#5374,.F.) ;
#7044=ORIENTED_EDGE('',*,*,#5336,.F.) ;
#7045=ORIENTED_EDGE('',*,*,#5329,.T.) ;
#7046=ORIENTED_EDGE('',*,*,#5326,.T.) ;
#7047=ORIENTED_EDGE('',*,*,#5322,.T.) ;
#7048=ORIENTED_EDGE('',*,*,#5334,.T.) ;
#7049=ORIENTED_EDGE('',*,*,#5339,.F.) ;
#7050=ORIENTED_EDGE('',*,*,#5375,.F.) ;
#7051=ORIENTED_EDGE('',*,*,#5298,.F.) ;
#7052=ORIENTED_EDGE('',*,*,#5286,.T.) ;
#7053=ORIENTED_EDGE('',*,*,#5282,.T.) ;
#7054=ORIENTED_EDGE('',*,*,#5291,.T.) ;
#7055=ORIENTED_EDGE('',*,*,#5363,.F.) ;
#7056=ORIENTED_EDGE('',*,*,#5379,.F.) ;
#7057=ORIENTED_EDGE('',*,*,#5306,.T.) ;
#7058=ORIENTED_EDGE('',*,*,#5368,.T.) ;
#7059=ORIENTED_EDGE('',*,*,#5361,.F.) ;
#7060=ORIENTED_EDGE('',*,*,#5380,.F.) ;
#7061=ORIENTED_EDGE('',*,*,#5307,.T.) ;
#7062=ORIENTED_EDGE('',*,*,#5379,.T.) ;
#7063=ORIENTED_EDGE('',*,*,#5358,.F.) ;
#7064=ORIENTED_EDGE('',*,*,#5381,.F.) ;
#7065=ORIENTED_EDGE('',*,*,#5308,.T.) ;
#7066=ORIENTED_EDGE('',*,*,#5380,.T.) ;
#7067=ORIENTED_EDGE('',*,*,#5355,.F.) ;
#7068=ORIENTED_EDGE('',*,*,#5365,.F.) ;
#7069=ORIENTED_EDGE('',*,*,#5309,.T.) ;
#7070=ORIENTED_EDGE('',*,*,#5381,.T.) ;
#9121=ADVANCED_FACE('',(#1185),#522,.F.) ;
#9122=ADVANCED_FACE('',(#1186),#523,.F.) ;
#9123=ADVANCED_FACE('',(#1187,#677),#819,.T.) ;
#9124=ADVANCED_FACE('',(#1188),#820,.T.) ;
#9125=ADVANCED_FACE('',(#1189),#821,.T.) ;
#9126=ADVANCED_FACE('',(#1190),#822,.T.) ;
#9127=ADVANCED_FACE('',(#1191,#678),#823,.F.) ;
#9128=ADVANCED_FACE('',(#1192),#524,.F.) ;
#9129=ADVANCED_FACE('',(#1193),#525,.F.) ;
#9130=ADVANCED_FACE('',(#1194,#679),#824,.F.) ;
#9131=ADVANCED_FACE('',(#1195,#680),#825,.F.) ;
#9132=ADVANCED_FACE('',(#1196),#826,.T.) ;
#9133=ADVANCED_FACE('',(#1197,#681),#827,.T.) ;
#9134=ADVANCED_FACE('',(#1198),#828,.T.) ;
#9135=ADVANCED_FACE('',(#1199),#829,.T.) ;
#9136=ADVANCED_FACE('',(#1200),#526,.F.) ;
#9137=ADVANCED_FACE('',(#1201),#527,.F.) ;
#9138=ADVANCED_FACE('',(#1202),#528,.T.) ;
#9139=ADVANCED_FACE('',(#1203),#331,.T.) ;
#9140=ADVANCED_FACE('',(#1204),#529,.T.) ;
#9141=ADVANCED_FACE('',(#1205),#332,.T.) ;
#9142=ADVANCED_FACE('',(#1206),#530,.T.) ;
#9143=ADVANCED_FACE('',(#1207),#333,.T.) ;
#9144=ADVANCED_FACE('',(#1208),#531,.T.) ;
#9145=ADVANCED_FACE('',(#1209),#334,.T.) ;
#9146=ADVANCED_FACE('',(#1210),#532,.T.) ;
#9147=ADVANCED_FACE('',(#1211),#830,.T.) ;
#9148=ADVANCED_FACE('',(#1212),#533,.T.) ;
#9149=ADVANCED_FACE('',(#1213),#831,.T.) ;
#9150=ADVANCED_FACE('',(#1214),#832,.T.) ;
#9151=ADVANCED_FACE('',(#1215),#833,.F.) ;
#9152=ADVANCED_FACE('',(#1216),#534,.F.) ;
#9153=ADVANCED_FACE('',(#1217),#834,.F.) ;
#9154=ADVANCED_FACE('',(#1218),#835,.F.) ;
#9155=ADVANCED_FACE('',(#1219),#836,.F.) ;
#9156=ADVANCED_FACE('',(#1220),#535,.F.) ;
#9157=ADVANCED_FACE('',(#1221),#837,.F.) ;
#9158=ADVANCED_FACE('',(#1222),#536,.T.) ;
#9159=ADVANCED_FACE('',(#1223),#838,.T.) ;
#9160=ADVANCED_FACE('',(#1224),#537,.T.) ;
#9161=ADVANCED_FACE('',(#1225),#839,.T.) ;
#9543=CLOSED_SHELL('',(#9121,#9122,#9123,#9124,#9125,#9126,#9127,#9128,
#9129,#9130,#9131,#9132,#9133,#9134,#9135,#9136,#9137,#9138,#9139,#9140,
#9141,#9142,#9143,#9144,#9145,#9146,#9147,#9148,#9149,#9150,#9151,#9152,
#9153,#9154,#9155,#9156,#9157,#9158,#9159,#9160,#9161)) ;
#9905=AXIS2_PLACEMENT_3D('',#14166,#11219,#11220) ;
#9906=AXIS2_PLACEMENT_3D('',#14167,#11221,#11222) ;
#9907=AXIS2_PLACEMENT_3D('',#14169,#11223,#11224) ;
#9908=AXIS2_PLACEMENT_3D('',#14172,#11226,#11227) ;
#9909=AXIS2_PLACEMENT_3D('',#14173,#11228,#11229) ;
#9910=AXIS2_PLACEMENT_3D('',#14175,#11230,#11231) ;
#9911=AXIS2_PLACEMENT_3D('',#14178,#11233,#11234) ;
#9912=AXIS2_PLACEMENT_3D('',#14179,#11235,#11236) ;
#9913=AXIS2_PLACEMENT_3D('',#14188,#11241,#11242) ;
#9914=AXIS2_PLACEMENT_3D('',#14198,#11248,#11249) ;
#9915=AXIS2_PLACEMENT_3D('',#14204,#11253,#11254) ;
#9916=AXIS2_PLACEMENT_3D('',#14206,#11256,#11257) ;
#9917=AXIS2_PLACEMENT_3D('',#14212,#11261,#11262) ;
#9918=AXIS2_PLACEMENT_3D('',#14214,#11263,#11264) ;
#9919=AXIS2_PLACEMENT_3D('',#14217,#11266,#11267) ;
#9920=AXIS2_PLACEMENT_3D('',#14218,#11268,#11269) ;
#9921=AXIS2_PLACEMENT_3D('',#14220,#11270,#11271) ;
#9922=AXIS2_PLACEMENT_3D('',#14223,#11273,#11274) ;
#9923=AXIS2_PLACEMENT_3D('',#14224,#11275,#11276) ;
#9924=AXIS2_PLACEMENT_3D('',#14227,#11277,#11278) ;
#9925=AXIS2_PLACEMENT_3D('',#14231,#11280,#11281) ;
#9926=AXIS2_PLACEMENT_3D('',#14235,#11283,#11284) ;
#9927=AXIS2_PLACEMENT_3D('',#14239,#11286,#11287) ;
#9928=AXIS2_PLACEMENT_3D('',#14244,#11290,#11291) ;
#9929=AXIS2_PLACEMENT_3D('',#14250,#11294,#11295) ;
#9930=AXIS2_PLACEMENT_3D('',#14254,#11297,#11298) ;
#9931=AXIS2_PLACEMENT_3D('',#14258,#11300,#11301) ;
#9932=AXIS2_PLACEMENT_3D('',#14260,#11303,#11304) ;
#9933=AXIS2_PLACEMENT_3D('',#14269,#11309,#11310) ;
#9934=AXIS2_PLACEMENT_3D('',#14275,#11314,#11315) ;
#9935=AXIS2_PLACEMENT_3D('',#14282,#11320,#11321) ;
#9936=AXIS2_PLACEMENT_3D('',#14284,#11323,#11324) ;
#9937=AXIS2_PLACEMENT_3D('',#14288,#11327,#11328) ;
#9938=AXIS2_PLACEMENT_3D('',#14290,#11329,#11330) ;
#9939=AXIS2_PLACEMENT_3D('',#14292,#11332,#11333) ;
#9940=AXIS2_PLACEMENT_3D('',#14295,#11335,#11336) ;
#9941=AXIS2_PLACEMENT_3D('',#14296,#11337,#11338) ;
#9942=AXIS2_PLACEMENT_3D('',#14299,#11339,#11340) ;
#9943=AXIS2_PLACEMENT_3D('',#14303,#11342,#11343) ;
#9944=AXIS2_PLACEMENT_3D('',#14305,#11345,#11346) ;
#9945=AXIS2_PLACEMENT_3D('',#14308,#11347,#11348) ;
#9946=AXIS2_PLACEMENT_3D('',#14309,#11349,#11350) ;
#9947=AXIS2_PLACEMENT_3D('',#14310,#11351,#11352) ;
#9948=AXIS2_PLACEMENT_3D('',#14311,#11353,#11354) ;
#9949=AXIS2_PLACEMENT_3D('',#14314,#11355,#11356) ;
#9950=AXIS2_PLACEMENT_3D('',#14317,#11359,#11360) ;
#9951=AXIS2_PLACEMENT_3D('',#14320,#11361,#11362) ;
#9952=AXIS2_PLACEMENT_3D('',#14321,#11363,#11364) ;
#9953=AXIS2_PLACEMENT_3D('',#14322,#11365,#11366) ;
#9954=AXIS2_PLACEMENT_3D('',#14323,#11367,#11368) ;
#9955=AXIS2_PLACEMENT_3D('',#14326,#11369,#11370) ;
#9956=AXIS2_PLACEMENT_3D('',#14329,#11373,#11374) ;
#9957=AXIS2_PLACEMENT_3D('',#14332,#11375,#11376) ;
#9958=AXIS2_PLACEMENT_3D('',#14333,#11377,#11378) ;
#9959=AXIS2_PLACEMENT_3D('',#14334,#11379,#11380) ;
#9960=AXIS2_PLACEMENT_3D('',#14335,#11381,#11382) ;
#9961=AXIS2_PLACEMENT_3D('',#14338,#11383,#11384) ;
#9962=AXIS2_PLACEMENT_3D('',#14341,#11387,#11388) ;
#9963=AXIS2_PLACEMENT_3D('',#14342,#11389,#11390) ;
#9964=AXIS2_PLACEMENT_3D('',#14343,#11391,#11392) ;
#9965=AXIS2_PLACEMENT_3D('',#14344,#11393,#11394) ;
#9966=AXIS2_PLACEMENT_3D('',#14347,#11397,#11398) ;
#9967=AXIS2_PLACEMENT_3D('',#14349,#11400,#11401) ;
#9968=AXIS2_PLACEMENT_3D('',#14351,#11403,#11404) ;
#9969=AXIS2_PLACEMENT_3D('',#14353,#11406,#11407) ;
#9970=AXIS2_PLACEMENT_3D('',#14354,#11408,#11409) ;
#9971=AXIS2_PLACEMENT_3D('',#14360,#11413,#11414) ;
#9972=AXIS2_PLACEMENT_3D('',#14363,#11416,#11417) ;
#9973=AXIS2_PLACEMENT_3D('',#14364,#11418,#11419) ;
#9974=AXIS2_PLACEMENT_3D('',#14366,#11421,#11422) ;
#9975=AXIS2_PLACEMENT_3D('',#14368,#11424,#11425) ;
#9976=AXIS2_PLACEMENT_3D('',#14372,#11428,#11429) ;
#9977=AXIS2_PLACEMENT_3D('',#14373,#11430,#11431) ;
#9978=AXIS2_PLACEMENT_3D('',#14374,#11432,#11433) ;
#9979=AXIS2_PLACEMENT_3D('',#14375,#11434,#11435) ;
#9980=AXIS2_PLACEMENT_3D('',#14377,#11437,#11438) ;
#9981=AXIS2_PLACEMENT_3D('',#14379,#11440,#11441) ;
#9982=AXIS2_PLACEMENT_3D('',#14381,#11443,#11444) ;
#11219=DIRECTION('axis',(0.,0.,1.)) ;
#11220=DIRECTION('refdir',(1.,0.,0.)) ;
#11221=DIRECTION('center_axis',(0.,1.,0.)) ;
#11222=DIRECTION('ref_axis',(1.,0.,0.)) ;
#11223=DIRECTION('center_axis',(0.,1.,0.)) ;
#11224=DIRECTION('ref_axis',(1.,0.,0.)) ;
#11225=DIRECTION('',(0.,1.,0.)) ;
#11226=DIRECTION('center_axis',(0.,-1.,0.)) ;
#11227=DIRECTION('ref_axis',(1.,0.,0.)) ;
#11228=DIRECTION('center_axis',(0.,1.,0.)) ;
#11229=DIRECTION('ref_axis',(1.,0.,0.)) ;
#11230=DIRECTION('center_axis',(0.,1.,0.)) ;
#11231=DIRECTION('ref_axis',(1.,0.,0.)) ;
#11232=DIRECTION('',(0.,1.,0.)) ;
#11233=DIRECTION('center_axis',(0.,-1.,0.)) ;
#11234=DIRECTION('ref_axis',(1.,0.,0.)) ;
#11235=DIRECTION('center_axis',(0.,1.,0.)) ;
#11236=DIRECTION('ref_axis',(0.,0.,1.)) ;
#11237=DIRECTION('',(-1.,0.,0.)) ;
#11238=DIRECTION('',(0.,0.,-1.)) ;
#11239=DIRECTION('',(-1.,0.,0.)) ;
#11240=DIRECTION('',(0.,0.,1.)) ;
#11241=DIRECTION('center_axis',(1.,0.,0.)) ;
#11242=DIRECTION('ref_axis',(0.,0.,-1.)) ;
#11243=DIRECTION('',(0.,1.,0.)) ;
#11244=DIRECTION('',(0.,0.,1.)) ;
#11245=DIRECTION('',(0.,1.,0.)) ;
#11246=DIRECTION('',(0.,0.,1.)) ;
#11247=DIRECTION('',(0.,1.,0.)) ;
#11248=DIRECTION('center_axis',(-1.,0.,0.)) ;
#11249=DIRECTION('ref_axis',(0.,0.,1.)) ;
#11250=DIRECTION('',(0.,-1.,0.)) ;
#11251=DIRECTION('',(0.,1.,0.)) ;
#11252=DIRECTION('',(0.,0.,-1.)) ;
#11253=DIRECTION('center_axis',(0.,0.,-1.)) ;
#11254=DIRECTION('ref_axis',(-1.,0.,0.)) ;
#11255=DIRECTION('',(1.,0.,0.)) ;
#11256=DIRECTION('center_axis',(0.,1.,0.)) ;
#11257=DIRECTION('ref_axis',(1.,0.,0.)) ;
#11258=DIRECTION('',(1.,0.,0.)) ;
#11259=DIRECTION('',(1.,0.,0.)) ;
#11260=DIRECTION('',(0.,0.,-1.)) ;
#11261=DIRECTION('center_axis',(0.,0.,1.)) ;
#11262=DIRECTION('ref_axis',(1.77635683940025E-15,-1.,0.)) ;
#11263=DIRECTION('center_axis',(0.,0.,1.)) ;
#11264=DIRECTION('ref_axis',(1.77635683940025E-15,-1.,0.)) ;
#11265=DIRECTION('',(0.,0.,1.)) ;
#11266=DIRECTION('center_axis',(0.,0.,1.)) ;
#11267=DIRECTION('ref_axis',(1.77635683940025E-15,-1.,0.)) ;
#11268=DIRECTION('center_axis',(0.,0.,1.)) ;
#11269=DIRECTION('ref_axis',(1.77635683940025E-15,-1.,0.)) ;
#11270=DIRECTION('center_axis',(0.,0.,1.)) ;
#11271=DIRECTION('ref_axis',(1.77635683940025E-15,-1.,0.)) ;
#11272=DIRECTION('',(0.,0.,1.)) ;
#11273=DIRECTION('center_axis',(0.,0.,1.)) ;
#11274=DIRECTION('ref_axis',(1.77635683940025E-15,-1.,0.)) ;
#11275=DIRECTION('center_axis',(0.,0.,1.)) ;
#11276=DIRECTION('ref_axis',(1.,0.,0.)) ;
#11277=DIRECTION('center_axis',(0.,0.,1.)) ;
#11278=DIRECTION('ref_axis',(-1.,-1.48029736616687E-15,0.)) ;
#11279=DIRECTION('',(0.,-1.,0.)) ;
#11280=DIRECTION('center_axis',(0.,0.,1.)) ;
#11281=DIRECTION('ref_axis',(-2.96059473233374E-15,1.,0.)) ;
#11282=DIRECTION('',(-1.,0.,0.)) ;
#11283=DIRECTION('center_axis',(0.,0.,1.)) ;
#11284=DIRECTION('ref_axis',(1.,1.48029736616687E-15,0.)) ;
#11285=DIRECTION('',(0.,1.,0.)) ;
#11286=DIRECTION('center_axis',(0.,0.,1.)) ;
#11287=DIRECTION('ref_axis',(2.96059473233374E-15,-1.,0.)) ;
#11288=DIRECTION('',(1.,0.,0.)) ;
#11289=DIRECTION('',(0.,1.,0.)) ;
#11290=DIRECTION('center_axis',(0.,0.,1.)) ;
#11291=DIRECTION('ref_axis',(1.,1.77635683940025E-15,0.)) ;
#11292=DIRECTION('',(0.,1.,0.)) ;
#11293=DIRECTION('',(-1.,0.,0.)) ;
#11294=DIRECTION('center_axis',(0.,0.,1.)) ;
#11295=DIRECTION('ref_axis',(1.,1.77635683940025E-15,0.)) ;
#11296=DIRECTION('',(-1.,0.,0.)) ;
#11297=DIRECTION('center_axis',(0.,0.,1.)) ;
#11298=DIRECTION('ref_axis',(-1.77635683940025E-15,1.,0.)) ;
#11299=DIRECTION('',(0.,-1.,0.)) ;
#11300=DIRECTION('center_axis',(0.,0.,1.)) ;
#11301=DIRECTION('ref_axis',(-1.,-1.77635683940025E-15,0.)) ;
#11302=DIRECTION('',(1.,0.,0.)) ;
#11303=DIRECTION('center_axis',(0.,1.,0.)) ;
#11304=DIRECTION('ref_axis',(1.,0.,0.)) ;
#11305=DIRECTION('',(1.,0.,0.)) ;
#11306=DIRECTION('',(0.,0.,-1.)) ;
#11307=DIRECTION('',(1.,0.,0.)) ;
#11308=DIRECTION('',(0.,0.,1.)) ;
#11309=DIRECTION('center_axis',(-1.,0.,0.)) ;
#11310=DIRECTION('ref_axis',(0.,0.,1.)) ;
#11311=DIRECTION('',(0.,-1.,0.)) ;
#11312=DIRECTION('',(0.,0.,1.)) ;
#11313=DIRECTION('',(0.,1.,0.)) ;
#11314=DIRECTION('center_axis',(0.,1.,0.)) ;
#11315=DIRECTION('ref_axis',(0.,0.,1.)) ;
#11316=DIRECTION('',(-1.,0.,0.)) ;
#11317=DIRECTION('',(0.,0.,1.)) ;
#11318=DIRECTION('',(0.,0.,-1.)) ;
#11319=DIRECTION('',(-1.,0.,0.)) ;
#11320=DIRECTION('center_axis',(0.,0.,-1.)) ;
#11321=DIRECTION('ref_axis',(-1.,0.,0.)) ;
#11322=DIRECTION('',(0.,1.,0.)) ;
#11323=DIRECTION('center_axis',(1.,0.,0.)) ;
#11324=DIRECTION('ref_axis',(0.,0.,-1.)) ;
#11325=DIRECTION('',(0.,1.,0.)) ;
#11326=DIRECTION('',(0.,0.,-1.)) ;
#11327=DIRECTION('center_axis',(0.,0.,1.)) ;
#11328=DIRECTION('ref_axis',(1.,1.77635683940025E-15,0.)) ;
#11329=DIRECTION('center_axis',(0.,0.,1.)) ;
#11330=DIRECTION('ref_axis',(1.,1.77635683940025E-15,0.)) ;
#11331=DIRECTION('',(0.,0.,1.)) ;
#11332=DIRECTION('center_axis',(0.,0.,1.)) ;
#11333=DIRECTION('ref_axis',(1.,1.77635683940025E-15,0.)) ;
#11334=DIRECTION('',(0.,0.,1.)) ;
#11335=DIRECTION('center_axis',(0.,0.,1.)) ;
#11336=DIRECTION('ref_axis',(1.,1.77635683940025E-15,0.)) ;
#11337=DIRECTION('center_axis',(0.,-1.,0.)) ;
#11338=DIRECTION('ref_axis',(-0.707106781186548,0.,0.707106781186548)) ;
#11339=DIRECTION('center_axis',(0.,-1.,0.)) ;
#11340=DIRECTION('ref_axis',(0.,0.,1.)) ;
#11341=DIRECTION('',(0.,-1.,0.)) ;
#11342=DIRECTION('center_axis',(0.,1.,0.)) ;
#11343=DIRECTION('ref_axis',(-1.,0.,0.)) ;
#11344=DIRECTION('',(0.,1.,0.)) ;
#11345=DIRECTION('center_axis',(0.,0.,1.)) ;
#11346=DIRECTION('ref_axis',(1.,0.,0.)) ;
#11347=DIRECTION('center_axis',(-1.,0.,0.)) ;
#11348=DIRECTION('ref_axis',(0.,-1.,0.)) ;
#11349=DIRECTION('center_axis',(0.,0.,-1.)) ;
#11350=DIRECTION('ref_axis',(-0.707106781186548,-0.707106781186548,0.)) ;
#11351=DIRECTION('center_axis',(0.,0.,1.)) ;
#11352=DIRECTION('ref_axis',(-0.707106781186547,-0.707106781186547,0.)) ;
#11353=DIRECTION('center_axis',(1.,0.,0.)) ;
#11354=DIRECTION('ref_axis',(0.,-0.70710678118656,0.707106781186535)) ;
#11355=DIRECTION('center_axis',(-1.,1.77635683940026E-14,0.)) ;
#11356=DIRECTION('ref_axis',(-1.77635683940026E-14,-1.,0.)) ;
#11357=DIRECTION('',(-1.,0.,0.)) ;
#11358=DIRECTION('',(1.,0.,0.)) ;
#11359=DIRECTION('center_axis',(0.,0.,1.)) ;
#11360=DIRECTION('ref_axis',(1.,0.,0.)) ;
#11361=DIRECTION('center_axis',(0.,-1.,0.)) ;
#11362=DIRECTION('ref_axis',(1.,0.,0.)) ;
#11363=DIRECTION('center_axis',(0.,0.,-1.)) ;
#11364=DIRECTION('ref_axis',(0.707106781186548,-0.707106781186548,0.)) ;
#11365=DIRECTION('center_axis',(0.,0.,1.)) ;
#11366=DIRECTION('ref_axis',(0.707106781186547,-0.707106781186547,0.)) ;
#11367=DIRECTION('center_axis',(0.,1.,0.)) ;
#11368=DIRECTION('ref_axis',(0.707106781186548,0.,0.707106781186548)) ;
#11369=DIRECTION('center_axis',(0.,-1.,0.)) ;
#11370=DIRECTION('ref_axis',(1.,0.,0.)) ;
#11371=DIRECTION('',(0.,-1.,0.)) ;
#11372=DIRECTION('',(0.,1.,0.)) ;
#11373=DIRECTION('center_axis',(0.,0.,1.)) ;
#11374=DIRECTION('ref_axis',(1.,0.,0.)) ;
#11375=DIRECTION('center_axis',(1.,0.,0.)) ;
#11376=DIRECTION('ref_axis',(0.,1.,0.)) ;
#11377=DIRECTION('center_axis',(0.,0.,-1.)) ;
#11378=DIRECTION('ref_axis',(0.707106781186548,0.707106781186548,0.)) ;
#11379=DIRECTION('center_axis',(0.,0.,1.)) ;
#11380=DIRECTION('ref_axis',(0.707106781186547,0.707106781186547,0.)) ;
#11381=DIRECTION('center_axis',(-1.,0.,0.)) ;
#11382=DIRECTION('ref_axis',(0.,0.70710678118656,0.707106781186535)) ;
#11383=DIRECTION('center_axis',(1.,-1.77635683940026E-14,0.)) ;
#11384=DIRECTION('ref_axis',(1.77635683940026E-14,1.,0.)) ;
#11385=DIRECTION('',(1.,0.,0.)) ;
#11386=DIRECTION('',(-1.,0.,0.)) ;
#11387=DIRECTION('center_axis',(0.,0.,1.)) ;
#11388=DIRECTION('ref_axis',(1.,0.,0.)) ;
#11389=DIRECTION('center_axis',(0.,0.,-1.)) ;
#11390=DIRECTION('ref_axis',(-0.707106781186548,0.707106781186548,0.)) ;
#11391=DIRECTION('center_axis',(0.,0.,1.)) ;
#11392=DIRECTION('ref_axis',(-0.707106781186547,0.707106781186547,0.)) ;
#11393=DIRECTION('center_axis',(0.,0.,1.)) ;
#11394=DIRECTION('ref_axis',(2.96059473233374E-15,-1.,0.)) ;
#11395=DIRECTION('',(0.,0.,1.)) ;
#11396=DIRECTION('',(0.,0.,1.)) ;
#11397=DIRECTION('center_axis',(0.,-1.,0.)) ;
#11398=DIRECTION('ref_axis',(1.,0.,0.)) ;
#11399=DIRECTION('',(0.,0.,1.)) ;
#11400=DIRECTION('center_axis',(0.,0.,1.)) ;
#11401=DIRECTION('ref_axis',(-1.,-1.48029736616687E-15,0.)) ;
#11402=DIRECTION('',(0.,0.,1.)) ;
#11403=DIRECTION('center_axis',(-1.,0.,0.)) ;
#11404=DIRECTION('ref_axis',(0.,-1.,0.)) ;
#11405=DIRECTION('',(0.,0.,1.)) ;
#11406=DIRECTION('center_axis',(0.,0.,1.)) ;
#11407=DIRECTION('ref_axis',(1.,0.,0.)) ;
#11408=DIRECTION('center_axis',(-1.,0.,0.)) ;
#11409=DIRECTION('ref_axis',(0.,-1.,0.)) ;
#11410=DIRECTION('',(0.,0.,1.)) ;
#11411=DIRECTION('',(0.,-1.,0.)) ;
#11412=DIRECTION('',(0.,0.,1.)) ;
#11413=DIRECTION('center_axis',(0.,0.,1.)) ;
#11414=DIRECTION('ref_axis',(-1.77635683940025E-15,1.,0.)) ;
#11415=DIRECTION('',(0.,0.,1.)) ;
#11416=DIRECTION('center_axis',(0.,0.,1.)) ;
#11417=DIRECTION('ref_axis',(-1.77635683940025E-15,1.,0.)) ;
#11418=DIRECTION('center_axis',(0.,1.,0.)) ;
#11419=DIRECTION('ref_axis',(-1.,0.,0.)) ;
#11420=DIRECTION('',(-1.,0.,0.)) ;
#11421=DIRECTION('center_axis',(1.,0.,0.)) ;
#11422=DIRECTION('ref_axis',(0.,1.,0.)) ;
#11423=DIRECTION('',(0.,1.,0.)) ;
#11424=DIRECTION('center_axis',(0.,-1.,0.)) ;
#11425=DIRECTION('ref_axis',(1.,0.,0.)) ;
#11426=DIRECTION('',(0.,0.,1.)) ;
#11427=DIRECTION('',(1.,0.,0.)) ;
#11428=DIRECTION('center_axis',(0.,0.,1.)) ;
#11429=DIRECTION('ref_axis',(-1.,-1.77635683940025E-15,0.)) ;
#11430=DIRECTION('center_axis',(0.,0.,1.)) ;
#11431=DIRECTION('ref_axis',(-1.,-1.77635683940025E-15,0.)) ;
#11432=DIRECTION('center_axis',(0.,0.,1.)) ;
#11433=DIRECTION('ref_axis',(1.,0.,0.)) ;
#11434=DIRECTION('center_axis',(0.,0.,1.)) ;
#11435=DIRECTION('ref_axis',(-2.96059473233374E-15,1.,0.)) ;
#11436=DIRECTION('',(0.,0.,1.)) ;
#11437=DIRECTION('center_axis',(0.,1.,0.)) ;
#11438=DIRECTION('ref_axis',(-1.,0.,0.)) ;
#11439=DIRECTION('',(0.,0.,1.)) ;
#11440=DIRECTION('center_axis',(0.,0.,1.)) ;
#11441=DIRECTION('ref_axis',(1.,1.48029736616687E-15,0.)) ;
#11442=DIRECTION('',(0.,0.,1.)) ;
#11443=DIRECTION('center_axis',(1.,0.,0.)) ;
#11444=DIRECTION('ref_axis',(0.,1.,0.)) ;
#14166=CARTESIAN_POINT('',(0.,0.,0.)) ;
#14167=CARTESIAN_POINT('Origin',(72.,-50.7,44.4)) ;
#14168=CARTESIAN_POINT('',(69.95,48.2,44.4)) ;
#14169=CARTESIAN_POINT('Origin',(72.,48.2,44.4)) ;
#14170=CARTESIAN_POINT('',(69.95,50.2,44.4)) ;
#14171=CARTESIAN_POINT('',(69.95,-50.7,44.4)) ;
#14172=CARTESIAN_POINT('Origin',(72.,50.2,44.4)) ;
#14173=CARTESIAN_POINT('Origin',(72.,-50.7,44.4)) ;
#14174=CARTESIAN_POINT('',(69.95,-50.2,44.4)) ;
#14175=CARTESIAN_POINT('Origin',(72.,-50.2,44.4)) ;
#14176=CARTESIAN_POINT('',(69.95,-48.2,44.4)) ;
#14177=CARTESIAN_POINT('',(69.95,-50.7,44.4)) ;
#14178=CARTESIAN_POINT('Origin',(72.,-48.2,44.4)) ;
#14179=CARTESIAN_POINT('Origin',(72.,-48.2,44.15)) ;
#14180=CARTESIAN_POINT('',(78.,-48.2,48.4)) ;
#14181=CARTESIAN_POINT('',(66.,-48.2,48.4)) ;
#14182=CARTESIAN_POINT('',(36.,-48.2,48.4)) ;
#14183=CARTESIAN_POINT('',(78.,-48.2,39.4)) ;
#14184=CARTESIAN_POINT('',(78.,-48.2,39.4)) ;
#14185=CARTESIAN_POINT('',(66.,-48.2,39.4)) ;
#14186=CARTESIAN_POINT('',(66.,-48.2,39.4)) ;
#14187=CARTESIAN_POINT('',(66.,-48.2,48.9)) ;
#14188=CARTESIAN_POINT('Origin',(78.,-50.2,48.9)) ;
#14189=CARTESIAN_POINT('',(78.,-49.35,48.4)) ;
#14190=CARTESIAN_POINT('',(78.,-25.1,48.4)) ;
#14191=CARTESIAN_POINT('',(78.,-49.35,43.4)) ;
#14192=CARTESIAN_POINT('',(78.,-49.35,43.4)) ;
#14193=CARTESIAN_POINT('',(78.,-50.2,43.4)) ;
#14194=CARTESIAN_POINT('',(78.,-25.1,43.4)) ;
#14195=CARTESIAN_POINT('',(78.,-50.2,39.4)) ;
#14196=CARTESIAN_POINT('',(78.,-50.2,39.4)) ;
#14197=CARTESIAN_POINT('',(78.,-50.2,39.4)) ;
#14198=CARTESIAN_POINT('Origin',(66.,-50.2,39.4)) ;
#14199=CARTESIAN_POINT('',(66.,-50.2,48.4)) ;
#14200=CARTESIAN_POINT('',(66.,-25.1,48.4)) ;
#14201=CARTESIAN_POINT('',(66.,-50.2,39.4)) ;
#14202=CARTESIAN_POINT('',(66.,-50.2,39.4)) ;
#14203=CARTESIAN_POINT('',(66.,-50.2,48.9)) ;
#14204=CARTESIAN_POINT('Origin',(78.,-50.2,39.4)) ;
#14205=CARTESIAN_POINT('',(66.,-50.2,39.4)) ;
#14206=CARTESIAN_POINT('Origin',(72.,-50.2,44.15)) ;
#14207=CARTESIAN_POINT('',(77.1902194281898,-50.2,48.4)) ;
#14208=CARTESIAN_POINT('',(36.,-50.2,48.4)) ;
#14209=CARTESIAN_POINT('',(77.1902194281898,-50.2,43.4)) ;
#14210=CARTESIAN_POINT('',(36.,-50.2,43.4)) ;
#14211=CARTESIAN_POINT('',(77.1902194281898,-50.2,43.4)) ;
#14212=CARTESIAN_POINT('Origin',(74.,-46.35,43.4)) ;
#14213=CARTESIAN_POINT('',(79.,-46.35,48.4)) ;
#14214=CARTESIAN_POINT('Origin',(74.,-46.35,48.4)) ;
#14215=CARTESIAN_POINT('',(79.,-46.35,43.4)) ;
#14216=CARTESIAN_POINT('',(79.,-46.35,43.4)) ;
#14217=CARTESIAN_POINT('Origin',(74.,-46.35,43.4)) ;
#14218=CARTESIAN_POINT('Origin',(74.,-46.35,43.4)) ;
#14219=CARTESIAN_POINT('',(74.,-51.35,43.4)) ;
#14220=CARTESIAN_POINT('Origin',(74.,-46.35,43.4)) ;
#14221=CARTESIAN_POINT('',(74.,-51.35,48.4)) ;
#14222=CARTESIAN_POINT('',(74.,-51.35,43.4)) ;
#14223=CARTESIAN_POINT('Origin',(74.,-46.35,48.4)) ;
#14224=CARTESIAN_POINT('Origin',(0.,0.,43.4)) ;
#14225=CARTESIAN_POINT('',(-80.,-46.35,43.4)) ;
#14226=CARTESIAN_POINT('',(-74.,-52.35,43.4)) ;
#14227=CARTESIAN_POINT('Origin',(-74.,-46.35,43.4)) ;
#14228=CARTESIAN_POINT('',(-80.,46.35,43.4)) ;
#14229=CARTESIAN_POINT('',(-80.,46.35,43.4)) ;
#14230=CARTESIAN_POINT('',(-74.,52.35,43.4)) ;
#14231=CARTESIAN_POINT('Origin',(-74.,46.35,43.4)) ;
#14232=CARTESIAN_POINT('',(74.,52.35,43.4)) ;
#14233=CARTESIAN_POINT('',(74.,52.35,43.4)) ;
#14234=CARTESIAN_POINT('',(80.,46.35,43.4)) ;
#14235=CARTESIAN_POINT('Origin',(74.,46.35,43.4)) ;
#14236=CARTESIAN_POINT('',(80.,-46.35,43.4)) ;
#14237=CARTESIAN_POINT('',(80.,-46.35,43.4)) ;
#14238=CARTESIAN_POINT('',(74.,-52.35,43.4)) ;
#14239=CARTESIAN_POINT('Origin',(74.,-46.35,43.4)) ;
#14240=CARTESIAN_POINT('',(-74.,-52.35,43.4)) ;
#14241=CARTESIAN_POINT('',(79.,46.35,43.4)) ;
#14242=CARTESIAN_POINT('',(79.,-23.175,43.4)) ;
#14243=CARTESIAN_POINT('',(78.,49.35,43.4)) ;
#14244=CARTESIAN_POINT('Origin',(74.,46.35,43.4)) ;
#14245=CARTESIAN_POINT('',(78.,50.2,43.4)) ;
#14246=CARTESIAN_POINT('',(78.,24.1,43.4)) ;
#14247=CARTESIAN_POINT('',(77.1902194281898,50.2,43.4)) ;
#14248=CARTESIAN_POINT('',(36.,50.2,43.4)) ;
#14249=CARTESIAN_POINT('',(74.,51.35,43.4)) ;
#14250=CARTESIAN_POINT('Origin',(74.,46.35,43.4)) ;
#14251=CARTESIAN_POINT('',(-74.,51.35,43.4)) ;
#14252=CARTESIAN_POINT('',(37.,51.35,43.4)) ;
#14253=CARTESIAN_POINT('',(-79.,46.35,43.4)) ;
#14254=CARTESIAN_POINT('Origin',(-74.,46.35,43.4)) ;
#14255=CARTESIAN_POINT('',(-79.,-46.35,43.4)) ;
#14256=CARTESIAN_POINT('',(-79.,23.175,43.4)) ;
#14257=CARTESIAN_POINT('',(-74.,-51.35,43.4)) ;
#14258=CARTESIAN_POINT('Origin',(-74.,-46.35,43.4)) ;
#14259=CARTESIAN_POINT('',(-37.,-51.35,43.4)) ;
#14260=CARTESIAN_POINT('Origin',(72.,48.2,44.15)) ;
#14261=CARTESIAN_POINT('',(66.,48.2,48.4)) ;
#14262=CARTESIAN_POINT('',(78.,48.2,48.4)) ;
#14263=CARTESIAN_POINT('',(36.,48.2,48.4)) ;
#14264=CARTESIAN_POINT('',(66.,48.2,39.4)) ;
#14265=CARTESIAN_POINT('',(66.,48.2,48.9)) ;
#14266=CARTESIAN_POINT('',(78.,48.2,39.4)) ;
#14267=CARTESIAN_POINT('',(66.,48.2,39.4)) ;
#14268=CARTESIAN_POINT('',(78.,48.2,39.4)) ;
#14269=CARTESIAN_POINT('Origin',(66.,48.2,39.4)) ;
#14270=CARTESIAN_POINT('',(66.,50.2,48.4)) ;
#14271=CARTESIAN_POINT('',(66.,24.1,48.4)) ;
#14272=CARTESIAN_POINT('',(66.,50.2,39.4)) ;
#14273=CARTESIAN_POINT('',(66.,50.2,48.9)) ;
#14274=CARTESIAN_POINT('',(66.,48.2,39.4)) ;
#14275=CARTESIAN_POINT('Origin',(72.,50.2,44.15)) ;
#14276=CARTESIAN_POINT('',(77.1902194281898,50.2,48.4)) ;
#14277=CARTESIAN_POINT('',(36.,50.2,48.4)) ;
#14278=CARTESIAN_POINT('',(77.1902194281898,50.2,43.4)) ;
#14279=CARTESIAN_POINT('',(78.,50.2,39.4)) ;
#14280=CARTESIAN_POINT('',(78.,50.2,39.4)) ;
#14281=CARTESIAN_POINT('',(66.,50.2,39.4)) ;
#14282=CARTESIAN_POINT('Origin',(78.,48.2,39.4)) ;
#14283=CARTESIAN_POINT('',(78.,48.2,39.4)) ;
#14284=CARTESIAN_POINT('Origin',(78.,48.2,48.9)) ;
#14285=CARTESIAN_POINT('',(78.,49.35,48.4)) ;
#14286=CARTESIAN_POINT('',(78.,24.1,48.4)) ;
#14287=CARTESIAN_POINT('',(78.,49.35,43.4)) ;
#14288=CARTESIAN_POINT('Origin',(74.,46.35,43.4)) ;
#14289=CARTESIAN_POINT('',(74.,51.35,48.4)) ;
#14290=CARTESIAN_POINT('Origin',(74.,46.35,48.4)) ;
#14291=CARTESIAN_POINT('',(74.,51.35,43.4)) ;
#14292=CARTESIAN_POINT('Origin',(74.,46.35,43.4)) ;
#14293=CARTESIAN_POINT('',(79.,46.35,48.4)) ;
#14294=CARTESIAN_POINT('',(79.,46.35,43.4)) ;
#14295=CARTESIAN_POINT('Origin',(74.,46.35,48.4)) ;
#14296=CARTESIAN_POINT('Origin',(-79.5,23.175,48.9)) ;
#14297=CARTESIAN_POINT('',(-79.5,46.35,49.4)) ;
#14298=CARTESIAN_POINT('',(-80.,46.35,48.9)) ;
#14299=CARTESIAN_POINT('Origin',(-79.5,46.35,48.9)) ;
#14300=CARTESIAN_POINT('',(-80.,-46.35,48.9)) ;
#14301=CARTESIAN_POINT('',(-80.,23.175,48.9)) ;
#14302=CARTESIAN_POINT('',(-79.5,-46.35,49.4)) ;
#14303=CARTESIAN_POINT('Origin',(-79.5,-46.35,48.9)) ;
#14304=CARTESIAN_POINT('',(-79.5,23.175,49.4)) ;
#14305=CARTESIAN_POINT('Origin',(-74.,-46.35,48.9)) ;
#14306=CARTESIAN_POINT('',(-74.,-52.35,48.9)) ;
#14307=CARTESIAN_POINT('',(-74.,-51.85,49.4)) ;
#14308=CARTESIAN_POINT('Origin',(-74.,-51.85,48.9)) ;
#14309=CARTESIAN_POINT('Origin',(-74.,-46.35,49.4)) ;
#14310=CARTESIAN_POINT('Origin',(-74.,-46.35,48.9)) ;
#14311=CARTESIAN_POINT('Origin',(-37.,-51.85,48.9)) ;
#14312=CARTESIAN_POINT('',(74.,-52.35,48.9)) ;
#14313=CARTESIAN_POINT('',(74.,-51.85,49.4)) ;
#14314=CARTESIAN_POINT('Origin',(74.,-51.85,48.9)) ;
#14315=CARTESIAN_POINT('',(-37.,-51.85,49.4)) ;
#14316=CARTESIAN_POINT('',(-37.,-52.35,48.9)) ;
#14317=CARTESIAN_POINT('Origin',(74.,-46.35,48.9)) ;
#14318=CARTESIAN_POINT('',(80.,-46.35,48.9)) ;
#14319=CARTESIAN_POINT('',(79.5,-46.35,49.4)) ;
#14320=CARTESIAN_POINT('Origin',(79.5,-46.35,48.9)) ;
#14321=CARTESIAN_POINT('Origin',(74.,-46.35,49.4)) ;
#14322=CARTESIAN_POINT('Origin',(74.,-46.35,48.9)) ;
#14323=CARTESIAN_POINT('Origin',(79.5,-23.175,48.9)) ;
#14324=CARTESIAN_POINT('',(80.,46.35,48.9)) ;
#14325=CARTESIAN_POINT('',(79.5,46.35,49.4)) ;
#14326=CARTESIAN_POINT('Origin',(79.5,46.35,48.9)) ;
#14327=CARTESIAN_POINT('',(79.5,-23.175,49.4)) ;
#14328=CARTESIAN_POINT('',(80.,-23.175,48.9)) ;
#14329=CARTESIAN_POINT('Origin',(74.,46.35,48.9)) ;
#14330=CARTESIAN_POINT('',(74.,52.35,48.9)) ;
#14331=CARTESIAN_POINT('',(74.,51.85,49.4)) ;
#14332=CARTESIAN_POINT('Origin',(74.,51.85,48.9)) ;
#14333=CARTESIAN_POINT('Origin',(74.,46.35,49.4)) ;
#14334=CARTESIAN_POINT('Origin',(74.,46.35,48.9)) ;
#14335=CARTESIAN_POINT('Origin',(37.,51.85,48.9)) ;
#14336=CARTESIAN_POINT('',(-74.,52.35,48.9)) ;
#14337=CARTESIAN_POINT('',(-74.,51.85,49.4)) ;
#14338=CARTESIAN_POINT('Origin',(-74.,51.85,48.9)) ;
#14339=CARTESIAN_POINT('',(37.,51.85,49.4)) ;
#14340=CARTESIAN_POINT('',(37.,52.35,48.9)) ;
#14341=CARTESIAN_POINT('Origin',(-74.,46.35,48.9)) ;
#14342=CARTESIAN_POINT('Origin',(-74.,46.35,49.4)) ;
#14343=CARTESIAN_POINT('Origin',(-74.,46.35,48.9)) ;
#14344=CARTESIAN_POINT('Origin',(74.,-46.35,43.4)) ;
#14345=CARTESIAN_POINT('',(74.,-52.35,43.4)) ;
#14346=CARTESIAN_POINT('',(80.,-46.35,43.4)) ;
#14347=CARTESIAN_POINT('Origin',(-74.,-52.35,43.4)) ;
#14348=CARTESIAN_POINT('',(-74.,-52.35,43.4)) ;
#14349=CARTESIAN_POINT('Origin',(-74.,-46.35,43.4)) ;
#14350=CARTESIAN_POINT('',(-80.,-46.35,43.4)) ;
#14351=CARTESIAN_POINT('Origin',(-80.,46.35,43.4)) ;
#14352=CARTESIAN_POINT('',(-80.,46.35,43.4)) ;
#14353=CARTESIAN_POINT('Origin',(0.,0.,49.4)) ;
#14354=CARTESIAN_POINT('Origin',(-79.,46.35,43.4)) ;
#14355=CARTESIAN_POINT('',(-79.,46.35,48.4)) ;
#14356=CARTESIAN_POINT('',(-79.,46.35,43.4)) ;
#14357=CARTESIAN_POINT('',(-79.,-46.35,48.4)) ;
#14358=CARTESIAN_POINT('',(-79.,46.35,48.4)) ;
#14359=CARTESIAN_POINT('',(-79.,-46.35,43.4)) ;
#14360=CARTESIAN_POINT('Origin',(-74.,46.35,43.4)) ;
#14361=CARTESIAN_POINT('',(-74.,51.35,48.4)) ;
#14362=CARTESIAN_POINT('',(-74.,51.35,43.4)) ;
#14363=CARTESIAN_POINT('Origin',(-74.,46.35,48.4)) ;
#14364=CARTESIAN_POINT('Origin',(74.,51.35,43.4)) ;
#14365=CARTESIAN_POINT('',(74.,51.35,48.4)) ;
#14366=CARTESIAN_POINT('Origin',(79.,-46.35,43.4)) ;
#14367=CARTESIAN_POINT('',(79.,-46.35,48.4)) ;
#14368=CARTESIAN_POINT('Origin',(-74.,-51.35,43.4)) ;
#14369=CARTESIAN_POINT('',(-74.,-51.35,48.4)) ;
#14370=CARTESIAN_POINT('',(-74.,-51.35,43.4)) ;
#14371=CARTESIAN_POINT('',(-74.,-51.35,48.4)) ;
#14372=CARTESIAN_POINT('Origin',(-74.,-46.35,43.4)) ;
#14373=CARTESIAN_POINT('Origin',(-74.,-46.35,48.4)) ;
#14374=CARTESIAN_POINT('Origin',(0.,0.,48.4)) ;
#14375=CARTESIAN_POINT('Origin',(-74.,46.35,43.4)) ;
#14376=CARTESIAN_POINT('',(-74.,52.35,43.4)) ;
#14377=CARTESIAN_POINT('Origin',(74.,52.35,43.4)) ;
#14378=CARTESIAN_POINT('',(74.,52.35,43.4)) ;
#14379=CARTESIAN_POINT('Origin',(74.,46.35,43.4)) ;
#14380=CARTESIAN_POINT('',(80.,46.35,43.4)) ;
#14381=CARTESIAN_POINT('Origin',(80.,-46.35,43.4)) ;
#18722=UNCERTAINTY_MEASURE_WITH_UNIT(LENGTH_MEASURE(0.01),#18758,
'DISTANCE_ACCURACY_VALUE',
'Maximum model space distance between geometric entities at asserted c
onnectivities') ;
#18738=UNCERTAINTY_MEASURE_WITH_UNIT(LENGTH_MEASURE(0.01),#18758,
'DISTANCE_ACCURACY_VALUE',
'Maximum model space distance between geometric entities at asserted c
onnectivities') ;
#18741=(
GEOMETRIC_REPRESENTATION_CONTEXT(3)
GLOBAL_UNCERTAINTY_ASSIGNED_CONTEXT((#18722))
GLOBAL_UNIT_ASSIGNED_CONTEXT((#18758,#18760,#18761))
REPRESENTATION_CONTEXT('','3D')
) ;
#18757=(
GEOMETRIC_REPRESENTATION_CONTEXT(3)
GLOBAL_UNCERTAINTY_ASSIGNED_CONTEXT((#18738))
GLOBAL_UNIT_ASSIGNED_CONTEXT((#18758,#18760,#18761))
REPRESENTATION_CONTEXT('','3D')
) ;
#18758=(
LENGTH_UNIT()
NAMED_UNIT(*)
SI_UNIT(.MILLI.,.METRE.)
) ;
#18760=(
NAMED_UNIT(*)
PLANE_ANGLE_UNIT()
SI_UNIT($,.RADIAN.)
) ;
#18761=(
NAMED_UNIT(*)
SI_UNIT($,.STERADIAN.)
SOLID_ANGLE_UNIT()
) ;
#18764=SHAPE_DEFINITION_REPRESENTATION(#18782,#18858) ;
#18782=PRODUCT_DEFINITION_SHAPE('',$,#18877) ;
#18858=SHAPE_REPRESENTATION('',(#9905),#18741) ;
#18874=PRODUCT_DEFINITION_CONTEXT('part definition',#18930,'design') ;
#18877=PRODUCT_DEFINITION('Lift Table Top 14 ga with Pivot Lugs',
'Lift Table Top 14 ga with Pivot Lugs',#18895,#18874) ;
#18895=PRODUCT_DEFINITION_FORMATION('',$,#18934) ;
#18930=APPLICATION_CONTEXT(
'Core Data for Automotive Mechanical Design Process') ;
#18931=PRODUCT_CONTEXT('part definition',#18930,'mechanical') ;
#18934=PRODUCT('Lift Table Top 14 ga with Pivot Lugs',
'Lift Table Top 14 ga with Pivot Lugs',$,(#18931)) ;
#18952=PRESENTATION_STYLE_ASSIGNMENT((#18970)) ;
#18970=SURFACE_STYLE_USAGE(.BOTH.,#18988) ;
#18988=SURFACE_SIDE_STYLE('',(#19006)) ;
#19006=SURFACE_STYLE_FILL_AREA(#19024) ;
#19024=FILL_AREA_STYLE(
'MAS-253 Metallic Sheet - Lift Table Top 14 ga with Pivot Lugs',(#19042)) ;
#19042=FILL_AREA_STYLE_COLOUR(
'MAS-253 Metallic Sheet - Lift Table Top 14 ga with Pivot Lugs',#19060) ;
#19060=COLOUR_RGB(
'MAS-253 Metallic Sheet - Lift Table Top 14 ga with Pivot Lugs', 0.31764706, 0.68627451, 0.89019608) ;
ENDSEC;
END-ISO-10303-21;
